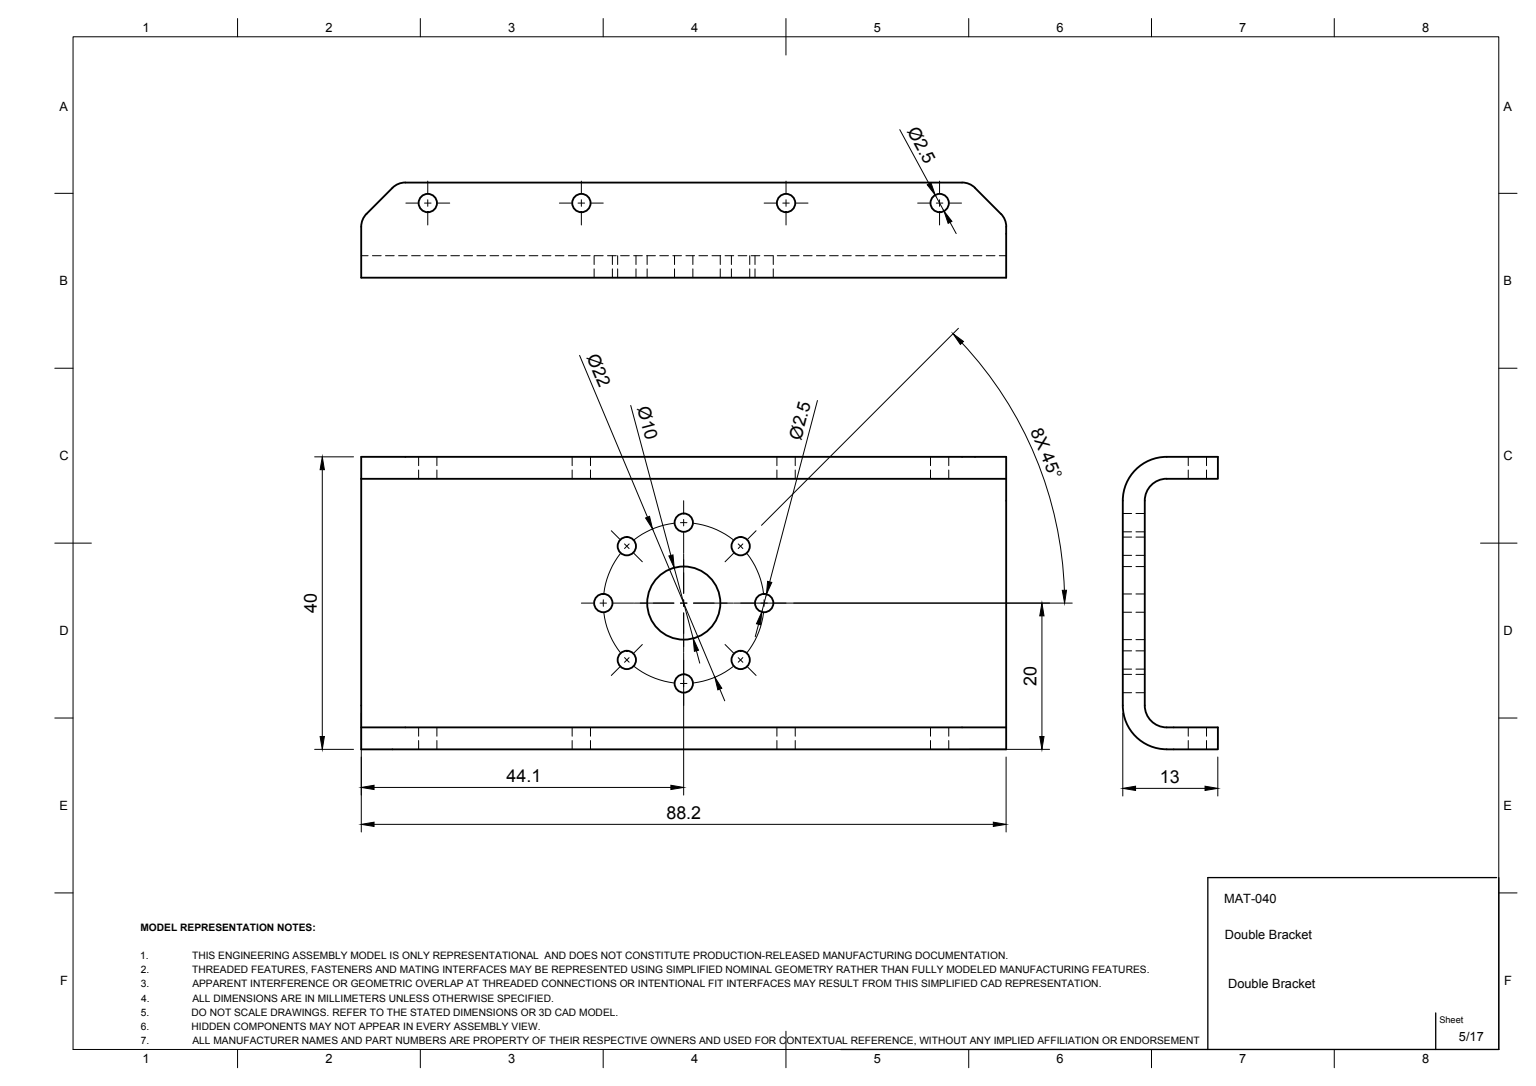
ISO-10303-21;
HEADER;
/* Generated by software containing ST-Developer
 * from STEP Tools, Inc. (www.steptools.com) 
 */

FILE_DESCRIPTION(
/* description */ ('STEP AP214'),
/* implementation_level */ '2;1');

FILE_NAME(
/* name */ 'Double Bracket.step',
/* time_stamp */ '2026-11-14T21:53:28-08:00',
/* author */ (''),
/* organization */ (''),
/* preprocessor_version */ 'ST-DEVELOPER v20.2',
/* originating_system */ 'Autodesk Translation Framework v15.17.0.0',
/* authorisation */ '');

FILE_SCHEMA (('AUTOMOTIVE_DESIGN { 1 0 10303 214 3 1 1 }'));
ENDSEC;

DATA;
#10=MECHANICAL_DESIGN_GEOMETRIC_PRESENTATION_REPRESENTATION('',(#318),#20176);
#294=SHAPE_REPRESENTATION_RELATIONSHIP('SRR','None',#20256,#306);
#306=ADVANCED_BREP_SHAPE_REPRESENTATION('',(#353),#20162);
#318=STYLED_ITEM('',(#20335),#353);
#353=MANIFOLD_SOLID_BREP('Body1',#10944);
#380=FACE_BOUND('',#1518,.T.);
#381=FACE_BOUND('',#1519,.T.);
#382=FACE_BOUND('',#1520,.T.);
#383=FACE_BOUND('',#1521,.T.);
#384=FACE_BOUND('',#1524,.T.);
#385=FACE_BOUND('',#1525,.T.);
#386=FACE_BOUND('',#1526,.T.);
#387=FACE_BOUND('',#1527,.T.);
#388=FACE_BOUND('',#1530,.T.);
#389=FACE_BOUND('',#1531,.T.);
#390=FACE_BOUND('',#1532,.T.);
#391=FACE_BOUND('',#1533,.T.);
#392=FACE_BOUND('',#1534,.T.);
#393=FACE_BOUND('',#1535,.T.);
#394=FACE_BOUND('',#1536,.T.);
#395=FACE_BOUND('',#1537,.T.);
#396=FACE_BOUND('',#1538,.T.);
#397=FACE_BOUND('',#1541,.T.);
#398=FACE_BOUND('',#1542,.T.);
#399=FACE_BOUND('',#1543,.T.);
#400=FACE_BOUND('',#1544,.T.);
#401=FACE_BOUND('',#1547,.T.);
#402=FACE_BOUND('',#1548,.T.);
#403=FACE_BOUND('',#1549,.T.);
#404=FACE_BOUND('',#1550,.T.);
#405=FACE_BOUND('',#1553,.T.);
#406=FACE_BOUND('',#1554,.T.);
#407=FACE_BOUND('',#1555,.T.);
#408=FACE_BOUND('',#1556,.T.);
#409=FACE_BOUND('',#1557,.T.);
#410=FACE_BOUND('',#1558,.T.);
#411=FACE_BOUND('',#1559,.T.);
#412=FACE_BOUND('',#1560,.T.);
#413=FACE_BOUND('',#1561,.T.);
#576=PLANE('',#11157);
#577=PLANE('',#11160);
#578=PLANE('',#11161);
#579=PLANE('',#11164);
#580=PLANE('',#11165);
#581=PLANE('',#11168);
#582=PLANE('',#11169);
#583=PLANE('',#11172);
#584=PLANE('',#11173);
#585=PLANE('',#11178);
#586=PLANE('',#11179);
#587=PLANE('',#11185);
#588=PLANE('',#11187);
#589=PLANE('',#11192);
#590=PLANE('',#11193);
#591=PLANE('',#11199);
#592=PLANE('',#11201);
#593=PLANE('',#11202);
#594=PLANE('',#11203);
#595=PLANE('',#11204);
#596=PLANE('',#11205);
#597=PLANE('',#11206);
#900=FACE_OUTER_BOUND('',#1492,.T.);
#901=FACE_OUTER_BOUND('',#1493,.T.);
#902=FACE_OUTER_BOUND('',#1494,.T.);
#903=FACE_OUTER_BOUND('',#1495,.T.);
#904=FACE_OUTER_BOUND('',#1496,.T.);
#905=FACE_OUTER_BOUND('',#1497,.T.);
#906=FACE_OUTER_BOUND('',#1498,.T.);
#907=FACE_OUTER_BOUND('',#1499,.T.);
#908=FACE_OUTER_BOUND('',#1500,.T.);
#909=FACE_OUTER_BOUND('',#1501,.T.);
#910=FACE_OUTER_BOUND('',#1502,.T.);
#911=FACE_OUTER_BOUND('',#1503,.T.);
#912=FACE_OUTER_BOUND('',#1504,.T.);
#913=FACE_OUTER_BOUND('',#1505,.T.);
#914=FACE_OUTER_BOUND('',#1506,.T.);
#915=FACE_OUTER_BOUND('',#1507,.T.);
#916=FACE_OUTER_BOUND('',#1508,.T.);
#917=FACE_OUTER_BOUND('',#1509,.T.);
#918=FACE_OUTER_BOUND('',#1510,.T.);
#919=FACE_OUTER_BOUND('',#1511,.T.);
#920=FACE_OUTER_BOUND('',#1512,.T.);
#921=FACE_OUTER_BOUND('',#1513,.T.);
#922=FACE_OUTER_BOUND('',#1514,.T.);
#923=FACE_OUTER_BOUND('',#1515,.T.);
#924=FACE_OUTER_BOUND('',#1516,.T.);
#925=FACE_OUTER_BOUND('',#1517,.T.);
#926=FACE_OUTER_BOUND('',#1522,.T.);
#927=FACE_OUTER_BOUND('',#1523,.T.);
#928=FACE_OUTER_BOUND('',#1528,.T.);
#929=FACE_OUTER_BOUND('',#1529,.T.);
#930=FACE_OUTER_BOUND('',#1539,.T.);
#931=FACE_OUTER_BOUND('',#1540,.T.);
#932=FACE_OUTER_BOUND('',#1545,.T.);
#933=FACE_OUTER_BOUND('',#1546,.T.);
#934=FACE_OUTER_BOUND('',#1551,.T.);
#935=FACE_OUTER_BOUND('',#1552,.T.);
#936=FACE_OUTER_BOUND('',#1562,.T.);
#937=FACE_OUTER_BOUND('',#1563,.T.);
#938=FACE_OUTER_BOUND('',#1564,.T.);
#939=FACE_OUTER_BOUND('',#1565,.T.);
#940=FACE_OUTER_BOUND('',#1566,.T.);
#941=FACE_OUTER_BOUND('',#1567,.T.);
#942=FACE_OUTER_BOUND('',#1568,.T.);
#943=FACE_OUTER_BOUND('',#1569,.T.);
#944=FACE_OUTER_BOUND('',#1570,.T.);
#945=FACE_OUTER_BOUND('',#1571,.T.);
#946=FACE_OUTER_BOUND('',#1572,.T.);
#947=FACE_OUTER_BOUND('',#1573,.T.);
#948=FACE_OUTER_BOUND('',#1574,.T.);
#949=FACE_OUTER_BOUND('',#1575,.T.);
#950=FACE_OUTER_BOUND('',#1576,.T.);
#1492=EDGE_LOOP('',(#7183,#7184,#7185,#7186));
#1493=EDGE_LOOP('',(#7187,#7188,#7189,#7190));
#1494=EDGE_LOOP('',(#7191,#7192,#7193,#7194));
#1495=EDGE_LOOP('',(#7195,#7196,#7197,#7198));
#1496=EDGE_LOOP('',(#7199,#7200,#7201,#7202));
#1497=EDGE_LOOP('',(#7203,#7204,#7205,#7206));
#1498=EDGE_LOOP('',(#7207,#7208,#7209,#7210));
#1499=EDGE_LOOP('',(#7211,#7212,#7213,#7214));
#1500=EDGE_LOOP('',(#7215,#7216,#7217,#7218));
#1501=EDGE_LOOP('',(#7219,#7220,#7221,#7222));
#1502=EDGE_LOOP('',(#7223,#7224,#7225,#7226));
#1503=EDGE_LOOP('',(#7227,#7228,#7229,#7230));
#1504=EDGE_LOOP('',(#7231,#7232,#7233,#7234));
#1505=EDGE_LOOP('',(#7235,#7236,#7237,#7238));
#1506=EDGE_LOOP('',(#7239,#7240,#7241,#7242));
#1507=EDGE_LOOP('',(#7243,#7244,#7245,#7246));
#1508=EDGE_LOOP('',(#7247,#7248,#7249,#7250));
#1509=EDGE_LOOP('',(#7251,#7252,#7253,#7254));
#1510=EDGE_LOOP('',(#7255,#7256,#7257,#7258));
#1511=EDGE_LOOP('',(#7259,#7260,#7261,#7262));
#1512=EDGE_LOOP('',(#7263,#7264,#7265,#7266));
#1513=EDGE_LOOP('',(#7267,#7268,#7269,#7270));
#1514=EDGE_LOOP('',(#7271,#7272,#7273,#7274));
#1515=EDGE_LOOP('',(#7275,#7276,#7277,#7278));
#1516=EDGE_LOOP('',(#7279,#7280,#7281,#7282));
#1517=EDGE_LOOP('',(#7283,#7284,#7285,#7286,#7287,#7288,#7289,#7290,#7291,
#7292));
#1518=EDGE_LOOP('',(#7293));
#1519=EDGE_LOOP('',(#7294));
#1520=EDGE_LOOP('',(#7295));
#1521=EDGE_LOOP('',(#7296));
#1522=EDGE_LOOP('',(#7297,#7298,#7299,#7300));
#1523=EDGE_LOOP('',(#7301,#7302,#7303,#7304,#7305,#7306,#7307,#7308,#7309,
#7310));
#1524=EDGE_LOOP('',(#7311));
#1525=EDGE_LOOP('',(#7312));
#1526=EDGE_LOOP('',(#7313));
#1527=EDGE_LOOP('',(#7314));
#1528=EDGE_LOOP('',(#7315,#7316,#7317,#7318));
#1529=EDGE_LOOP('',(#7319,#7320,#7321,#7322));
#1530=EDGE_LOOP('',(#7323));
#1531=EDGE_LOOP('',(#7324));
#1532=EDGE_LOOP('',(#7325));
#1533=EDGE_LOOP('',(#7326));
#1534=EDGE_LOOP('',(#7327));
#1535=EDGE_LOOP('',(#7328));
#1536=EDGE_LOOP('',(#7329));
#1537=EDGE_LOOP('',(#7330));
#1538=EDGE_LOOP('',(#7331));
#1539=EDGE_LOOP('',(#7332,#7333,#7334,#7335));
#1540=EDGE_LOOP('',(#7336,#7337,#7338,#7339,#7340,#7341,#7342,#7343,#7344,
#7345));
#1541=EDGE_LOOP('',(#7346));
#1542=EDGE_LOOP('',(#7347));
#1543=EDGE_LOOP('',(#7348));
#1544=EDGE_LOOP('',(#7349));
#1545=EDGE_LOOP('',(#7350,#7351,#7352,#7353));
#1546=EDGE_LOOP('',(#7354,#7355,#7356,#7357,#7358,#7359,#7360,#7361,#7362,
#7363));
#1547=EDGE_LOOP('',(#7364));
#1548=EDGE_LOOP('',(#7365));
#1549=EDGE_LOOP('',(#7366));
#1550=EDGE_LOOP('',(#7367));
#1551=EDGE_LOOP('',(#7368,#7369,#7370,#7371));
#1552=EDGE_LOOP('',(#7372,#7373,#7374,#7375));
#1553=EDGE_LOOP('',(#7376));
#1554=EDGE_LOOP('',(#7377));
#1555=EDGE_LOOP('',(#7378));
#1556=EDGE_LOOP('',(#7379));
#1557=EDGE_LOOP('',(#7380));
#1558=EDGE_LOOP('',(#7381));
#1559=EDGE_LOOP('',(#7382));
#1560=EDGE_LOOP('',(#7383));
#1561=EDGE_LOOP('',(#7384));
#1562=EDGE_LOOP('',(#7385,#7386,#7387,#7388));
#1563=EDGE_LOOP('',(#7389,#7390,#7391,#7392));
#1564=EDGE_LOOP('',(#7393,#7394,#7395,#7396));
#1565=EDGE_LOOP('',(#7397,#7398,#7399,#7400));
#1566=EDGE_LOOP('',(#7401,#7402,#7403,#7404));
#1567=EDGE_LOOP('',(#7405,#7406,#7407,#7408));
#1568=EDGE_LOOP('',(#7409,#7410,#7411,#7412));
#1569=EDGE_LOOP('',(#7413,#7414,#7415,#7416));
#1570=EDGE_LOOP('',(#7417,#7418,#7419,#7420));
#1571=EDGE_LOOP('',(#7421,#7422,#7423,#7424));
#1572=EDGE_LOOP('',(#7425,#7426,#7427,#7428));
#1573=EDGE_LOOP('',(#7429,#7430,#7431,#7432));
#1574=EDGE_LOOP('',(#7433,#7434,#7435,#7436));
#1575=EDGE_LOOP('',(#7437,#7438,#7439,#7440));
#1576=EDGE_LOOP('',(#7441,#7442,#7443,#7444));
#2280=LINE('',#15428,#3268);
#2281=LINE('',#15434,#3269);
#2282=LINE('',#15440,#3270);
#2283=LINE('',#15446,#3271);
#2284=LINE('',#15452,#3272);
#2285=LINE('',#15458,#3273);
#2286=LINE('',#15464,#3274);
#2287=LINE('',#15470,#3275);
#2288=LINE('',#15476,#3276);
#2289=LINE('',#15482,#3277);
#2290=LINE('',#15488,#3278);
#2291=LINE('',#15494,#3279);
#2292=LINE('',#15500,#3280);
#2293=LINE('',#15506,#3281);
#2294=LINE('',#15512,#3282);
#2295=LINE('',#15518,#3283);
#2296=LINE('',#15524,#3284);
#2297=LINE('',#15529,#3285);
#2298=LINE('',#15533,#3286);
#2299=LINE('',#15537,#3287);
#2300=LINE('',#15539,#3288);
#2301=LINE('',#15540,#3289);
#2302=LINE('',#15544,#3290);
#2303=LINE('',#15548,#3291);
#2304=LINE('',#15552,#3292);
#2305=LINE('',#15554,#3293);
#2306=LINE('',#15555,#3294);
#2307=LINE('',#15559,#3295);
#2308=LINE('',#15564,#3296);
#2309=LINE('',#15566,#3297);
#2310=LINE('',#15567,#3298);
#2311=LINE('',#15571,#3299);
#2312=LINE('',#15575,#3300);
#2313=LINE('',#15578,#3301);
#2314=LINE('',#15579,#3302);
#2315=LINE('',#15583,#3303);
#2316=LINE('',#15585,#3304);
#2317=LINE('',#15587,#3305);
#2318=LINE('',#15591,#3306);
#2319=LINE('',#15595,#3307);
#2320=LINE('',#15600,#3308);
#2321=LINE('',#15601,#3309);
#2322=LINE('',#15602,#3310);
#2323=LINE('',#15607,#3311);
#2324=LINE('',#15612,#3312);
#2325=LINE('',#15615,#3313);
#2326=LINE('',#15616,#3314);
#2327=LINE('',#15618,#3315);
#2328=LINE('',#15620,#3316);
#2329=LINE('',#15622,#3317);
#2330=LINE('',#15627,#3318);
#2331=LINE('',#15631,#3319);
#2332=LINE('',#15635,#3320);
#2333=LINE('',#15638,#3321);
#2334=LINE('',#15641,#3322);
#2335=LINE('',#15643,#3323);
#2336=LINE('',#15644,#3324);
#2337=LINE('',#15648,#3325);
#2338=LINE('',#15650,#3326);
#2339=LINE('',#15652,#3327);
#2340=LINE('',#15656,#3328);
#2341=LINE('',#15660,#3329);
#2342=LINE('',#15662,#3330);
#2343=LINE('',#15665,#3331);
#2344=LINE('',#15667,#3332);
#2345=LINE('',#15669,#3333);
#2346=LINE('',#15670,#3334);
#2347=LINE('',#15672,#3335);
#2348=LINE('',#15673,#3336);
#2349=LINE('',#15675,#3337);
#2350=LINE('',#15676,#3338);
#2351=LINE('',#15678,#3339);
#2352=LINE('',#15679,#3340);
#3268=VECTOR('',#12222,1.25);
#3269=VECTOR('',#12229,1.25);
#3270=VECTOR('',#12236,1.25);
#3271=VECTOR('',#12243,1.25);
#3272=VECTOR('',#12250,1.25);
#3273=VECTOR('',#12257,1.25);
#3274=VECTOR('',#12264,1.25);
#3275=VECTOR('',#12271,1.25);
#3276=VECTOR('',#12278,1.25);
#3277=VECTOR('',#12285,1.25);
#3278=VECTOR('',#12292,1.25);
#3279=VECTOR('',#12299,1.25);
#3280=VECTOR('',#12306,1.25);
#3281=VECTOR('',#12313,1.25);
#3282=VECTOR('',#12320,1.25);
#3283=VECTOR('',#12327,1.25);
#3284=VECTOR('',#12334,5.);
#3285=VECTOR('',#12339,1000.);
#3286=VECTOR('',#12342,1000.);
#3287=VECTOR('',#12347,1000.);
#3288=VECTOR('',#12348,1000.);
#3289=VECTOR('',#12349,1000.);
#3290=VECTOR('',#12352,1000.);
#3291=VECTOR('',#12355,1000.);
#3292=VECTOR('',#12360,1000.);
#3293=VECTOR('',#12361,1000.);
#3294=VECTOR('',#12362,1000.);
#3295=VECTOR('',#12365,1000.);
#3296=VECTOR('',#12372,1000.);
#3297=VECTOR('',#12373,1000.);
#3298=VECTOR('',#12374,1000.);
#3299=VECTOR('',#12377,1000.);
#3300=VECTOR('',#12380,1000.);
#3301=VECTOR('',#12385,1000.);
#3302=VECTOR('',#12386,1000.);
#3303=VECTOR('',#12389,1000.);
#3304=VECTOR('',#12392,1000.);
#3305=VECTOR('',#12393,1000.);
#3306=VECTOR('',#12396,1000.);
#3307=VECTOR('',#12399,1000.);
#3308=VECTOR('',#12404,1000.);
#3309=VECTOR('',#12405,1000.);
#3310=VECTOR('',#12406,1000.);
#3311=VECTOR('',#12411,1000.);
#3312=VECTOR('',#12416,1000.);
#3313=VECTOR('',#12419,1000.);
#3314=VECTOR('',#12420,1000.);
#3315=VECTOR('',#12423,1000.);
#3316=VECTOR('',#12426,1000.);
#3317=VECTOR('',#12429,1000.);
#3318=VECTOR('',#12434,1000.);
#3319=VECTOR('',#12437,1000.);
#3320=VECTOR('',#12440,1000.);
#3321=VECTOR('',#12443,1000.);
#3322=VECTOR('',#12446,1000.);
#3323=VECTOR('',#12447,1000.);
#3324=VECTOR('',#12448,1000.);
#3325=VECTOR('',#12451,1000.);
#3326=VECTOR('',#12454,1000.);
#3327=VECTOR('',#12455,1000.);
#3328=VECTOR('',#12458,1000.);
#3329=VECTOR('',#12465,1000.);
#3330=VECTOR('',#12468,1000.);
#3331=VECTOR('',#12473,1000.);
#3332=VECTOR('',#12476,1000.);
#3333=VECTOR('',#12479,1000.);
#3334=VECTOR('',#12480,1000.);
#3335=VECTOR('',#12483,1000.);
#3336=VECTOR('',#12484,1000.);
#3337=VECTOR('',#12487,1000.);
#3338=VECTOR('',#12488,1000.);
#3339=VECTOR('',#12491,1000.);
#3340=VECTOR('',#12492,1000.);
#4256=CIRCLE('',#11107,1.25);
#4257=CIRCLE('',#11108,1.25);
#4258=CIRCLE('',#11110,1.25);
#4259=CIRCLE('',#11111,1.25);
#4260=CIRCLE('',#11113,1.25);
#4261=CIRCLE('',#11114,1.25);
#4262=CIRCLE('',#11116,1.25);
#4263=CIRCLE('',#11117,1.25);
#4264=CIRCLE('',#11119,1.25);
#4265=CIRCLE('',#11120,1.25);
#4266=CIRCLE('',#11122,1.25);
#4267=CIRCLE('',#11123,1.25);
#4268=CIRCLE('',#11125,1.25);
#4269=CIRCLE('',#11126,1.25);
#4270=CIRCLE('',#11128,1.25);
#4271=CIRCLE('',#11129,1.25);
#4272=CIRCLE('',#11131,1.24999999999999);
#4273=CIRCLE('',#11132,1.25);
#4274=CIRCLE('',#11134,1.24999999999999);
#4275=CIRCLE('',#11135,1.25);
#4276=CIRCLE('',#11137,1.24999999999999);
#4277=CIRCLE('',#11138,1.25);
#4278=CIRCLE('',#11140,1.24999999999999);
#4279=CIRCLE('',#11141,1.25);
#4280=CIRCLE('',#11143,1.24999999999999);
#4281=CIRCLE('',#11144,1.25);
#4282=CIRCLE('',#11146,1.25);
#4283=CIRCLE('',#11147,1.25);
#4284=CIRCLE('',#11149,1.25000000000001);
#4285=CIRCLE('',#11150,1.25);
#4286=CIRCLE('',#11152,1.25);
#4287=CIRCLE('',#11153,1.25);
#4288=CIRCLE('',#11155,5.);
#4289=CIRCLE('',#11156,5.);
#4290=CIRCLE('',#11158,3.);
#4291=CIRCLE('',#11159,6.);
#4292=CIRCLE('',#11162,3.);
#4293=CIRCLE('',#11163,6.);
#4294=CIRCLE('',#11166,3.);
#4295=CIRCLE('',#11167,6.);
#4296=CIRCLE('',#11170,3.);
#4297=CIRCLE('',#11171,6.);
#4298=CIRCLE('',#11174,2.5);
#4299=CIRCLE('',#11175,2.5);
#4300=CIRCLE('',#11176,2.5);
#4301=CIRCLE('',#11177,2.5);
#4302=CIRCLE('',#11180,2.5);
#4303=CIRCLE('',#11181,2.5);
#4304=CIRCLE('',#11182,2.5);
#4305=CIRCLE('',#11183,2.5);
#4306=CIRCLE('',#11188,2.5);
#4307=CIRCLE('',#11189,2.5);
#4308=CIRCLE('',#11190,2.5);
#4309=CIRCLE('',#11191,2.5);
#4310=CIRCLE('',#11194,2.5);
#4311=CIRCLE('',#11195,2.5);
#4312=CIRCLE('',#11196,2.5);
#4313=CIRCLE('',#11197,2.5);
#4727=VERTEX_POINT('',#15425);
#4728=VERTEX_POINT('',#15427);
#4729=VERTEX_POINT('',#15431);
#4730=VERTEX_POINT('',#15433);
#4731=VERTEX_POINT('',#15437);
#4732=VERTEX_POINT('',#15439);
#4733=VERTEX_POINT('',#15443);
#4734=VERTEX_POINT('',#15445);
#4735=VERTEX_POINT('',#15449);
#4736=VERTEX_POINT('',#15451);
#4737=VERTEX_POINT('',#15455);
#4738=VERTEX_POINT('',#15457);
#4739=VERTEX_POINT('',#15461);
#4740=VERTEX_POINT('',#15463);
#4741=VERTEX_POINT('',#15467);
#4742=VERTEX_POINT('',#15469);
#4743=VERTEX_POINT('',#15473);
#4744=VERTEX_POINT('',#15475);
#4745=VERTEX_POINT('',#15479);
#4746=VERTEX_POINT('',#15481);
#4747=VERTEX_POINT('',#15485);
#4748=VERTEX_POINT('',#15487);
#4749=VERTEX_POINT('',#15491);
#4750=VERTEX_POINT('',#15493);
#4751=VERTEX_POINT('',#15497);
#4752=VERTEX_POINT('',#15499);
#4753=VERTEX_POINT('',#15503);
#4754=VERTEX_POINT('',#15505);
#4755=VERTEX_POINT('',#15509);
#4756=VERTEX_POINT('',#15511);
#4757=VERTEX_POINT('',#15515);
#4758=VERTEX_POINT('',#15517);
#4759=VERTEX_POINT('',#15521);
#4760=VERTEX_POINT('',#15523);
#4761=VERTEX_POINT('',#15527);
#4762=VERTEX_POINT('',#15528);
#4763=VERTEX_POINT('',#15530);
#4764=VERTEX_POINT('',#15532);
#4765=VERTEX_POINT('',#15536);
#4766=VERTEX_POINT('',#15538);
#4767=VERTEX_POINT('',#15542);
#4768=VERTEX_POINT('',#15543);
#4769=VERTEX_POINT('',#15545);
#4770=VERTEX_POINT('',#15547);
#4771=VERTEX_POINT('',#15551);
#4772=VERTEX_POINT('',#15553);
#4773=VERTEX_POINT('',#15557);
#4774=VERTEX_POINT('',#15558);
#4775=VERTEX_POINT('',#15563);
#4776=VERTEX_POINT('',#15565);
#4777=VERTEX_POINT('',#15569);
#4778=VERTEX_POINT('',#15570);
#4779=VERTEX_POINT('',#15572);
#4780=VERTEX_POINT('',#15574);
#4781=VERTEX_POINT('',#15581);
#4782=VERTEX_POINT('',#15582);
#4783=VERTEX_POINT('',#15586);
#4784=VERTEX_POINT('',#15588);
#4785=VERTEX_POINT('',#15590);
#4786=VERTEX_POINT('',#15592);
#4787=VERTEX_POINT('',#15594);
#4788=VERTEX_POINT('',#15598);
#4789=VERTEX_POINT('',#15599);
#4790=VERTEX_POINT('',#15604);
#4791=VERTEX_POINT('',#15606);
#4792=VERTEX_POINT('',#15609);
#4793=VERTEX_POINT('',#15611);
#4794=VERTEX_POINT('',#15613);
#4795=VERTEX_POINT('',#15624);
#4796=VERTEX_POINT('',#15626);
#4797=VERTEX_POINT('',#15628);
#4798=VERTEX_POINT('',#15630);
#4799=VERTEX_POINT('',#15632);
#4800=VERTEX_POINT('',#15634);
#4801=VERTEX_POINT('',#15636);
#4802=VERTEX_POINT('',#15640);
#4803=VERTEX_POINT('',#15642);
#4804=VERTEX_POINT('',#15646);
#4805=VERTEX_POINT('',#15647);
#4806=VERTEX_POINT('',#15651);
#4807=VERTEX_POINT('',#15653);
#4808=VERTEX_POINT('',#15655);
#5694=EDGE_CURVE('',#4727,#4727,#4256,.T.);
#5695=EDGE_CURVE('',#4727,#4728,#2280,.T.);
#5696=EDGE_CURVE('',#4728,#4728,#4257,.T.);
#5697=EDGE_CURVE('',#4729,#4729,#4258,.T.);
#5698=EDGE_CURVE('',#4729,#4730,#2281,.T.);
#5699=EDGE_CURVE('',#4730,#4730,#4259,.T.);
#5700=EDGE_CURVE('',#4731,#4731,#4260,.T.);
#5701=EDGE_CURVE('',#4731,#4732,#2282,.T.);
#5702=EDGE_CURVE('',#4732,#4732,#4261,.T.);
#5703=EDGE_CURVE('',#4733,#4733,#4262,.T.);
#5704=EDGE_CURVE('',#4733,#4734,#2283,.T.);
#5705=EDGE_CURVE('',#4734,#4734,#4263,.T.);
#5706=EDGE_CURVE('',#4735,#4735,#4264,.T.);
#5707=EDGE_CURVE('',#4735,#4736,#2284,.T.);
#5708=EDGE_CURVE('',#4736,#4736,#4265,.T.);
#5709=EDGE_CURVE('',#4737,#4737,#4266,.T.);
#5710=EDGE_CURVE('',#4737,#4738,#2285,.T.);
#5711=EDGE_CURVE('',#4738,#4738,#4267,.T.);
#5712=EDGE_CURVE('',#4739,#4739,#4268,.T.);
#5713=EDGE_CURVE('',#4739,#4740,#2286,.T.);
#5714=EDGE_CURVE('',#4740,#4740,#4269,.T.);
#5715=EDGE_CURVE('',#4741,#4741,#4270,.T.);
#5716=EDGE_CURVE('',#4741,#4742,#2287,.T.);
#5717=EDGE_CURVE('',#4742,#4742,#4271,.T.);
#5718=EDGE_CURVE('',#4743,#4743,#4272,.T.);
#5719=EDGE_CURVE('',#4743,#4744,#2288,.T.);
#5720=EDGE_CURVE('',#4744,#4744,#4273,.T.);
#5721=EDGE_CURVE('',#4745,#4745,#4274,.T.);
#5722=EDGE_CURVE('',#4745,#4746,#2289,.T.);
#5723=EDGE_CURVE('',#4746,#4746,#4275,.T.);
#5724=EDGE_CURVE('',#4747,#4747,#4276,.T.);
#5725=EDGE_CURVE('',#4747,#4748,#2290,.T.);
#5726=EDGE_CURVE('',#4748,#4748,#4277,.T.);
#5727=EDGE_CURVE('',#4749,#4749,#4278,.T.);
#5728=EDGE_CURVE('',#4749,#4750,#2291,.T.);
#5729=EDGE_CURVE('',#4750,#4750,#4279,.T.);
#5730=EDGE_CURVE('',#4751,#4751,#4280,.T.);
#5731=EDGE_CURVE('',#4751,#4752,#2292,.T.);
#5732=EDGE_CURVE('',#4752,#4752,#4281,.T.);
#5733=EDGE_CURVE('',#4753,#4753,#4282,.T.);
#5734=EDGE_CURVE('',#4753,#4754,#2293,.T.);
#5735=EDGE_CURVE('',#4754,#4754,#4283,.T.);
#5736=EDGE_CURVE('',#4755,#4755,#4284,.T.);
#5737=EDGE_CURVE('',#4755,#4756,#2294,.T.);
#5738=EDGE_CURVE('',#4756,#4756,#4285,.T.);
#5739=EDGE_CURVE('',#4757,#4757,#4286,.T.);
#5740=EDGE_CURVE('',#4757,#4758,#2295,.T.);
#5741=EDGE_CURVE('',#4758,#4758,#4287,.T.);
#5742=EDGE_CURVE('',#4759,#4759,#4288,.T.);
#5743=EDGE_CURVE('',#4759,#4760,#2296,.T.);
#5744=EDGE_CURVE('',#4760,#4760,#4289,.T.);
#5745=EDGE_CURVE('',#4761,#4762,#2297,.T.);
#5746=EDGE_CURVE('',#4763,#4761,#4290,.T.);
#5747=EDGE_CURVE('',#4764,#4763,#2298,.T.);
#5748=EDGE_CURVE('',#4764,#4762,#4291,.T.);
#5749=EDGE_CURVE('',#4761,#4765,#2299,.T.);
#5750=EDGE_CURVE('',#4762,#4766,#2300,.T.);
#5751=EDGE_CURVE('',#4766,#4765,#2301,.T.);
#5752=EDGE_CURVE('',#4767,#4768,#2302,.T.);
#5753=EDGE_CURVE('',#4767,#4769,#4292,.T.);
#5754=EDGE_CURVE('',#4770,#4769,#2303,.T.);
#5755=EDGE_CURVE('',#4768,#4770,#4293,.T.);
#5756=EDGE_CURVE('',#4771,#4768,#2304,.T.);
#5757=EDGE_CURVE('',#4771,#4772,#2305,.T.);
#5758=EDGE_CURVE('',#4772,#4767,#2306,.T.);
#5759=EDGE_CURVE('',#4773,#4774,#2307,.T.);
#5760=EDGE_CURVE('',#4765,#4773,#4294,.T.);
#5761=EDGE_CURVE('',#4766,#4774,#4295,.T.);
#5762=EDGE_CURVE('',#4774,#4775,#2308,.T.);
#5763=EDGE_CURVE('',#4775,#4776,#2309,.T.);
#5764=EDGE_CURVE('',#4773,#4776,#2310,.T.);
#5765=EDGE_CURVE('',#4777,#4778,#2311,.T.);
#5766=EDGE_CURVE('',#4777,#4779,#4296,.T.);
#5767=EDGE_CURVE('',#4780,#4779,#2312,.T.);
#5768=EDGE_CURVE('',#4778,#4780,#4297,.T.);
#5769=EDGE_CURVE('',#4769,#4777,#2313,.T.);
#5770=EDGE_CURVE('',#4770,#4778,#2314,.T.);
#5771=EDGE_CURVE('',#4781,#4782,#2315,.T.);
#5772=EDGE_CURVE('',#4782,#4775,#4298,.T.);
#5773=EDGE_CURVE('',#4774,#4780,#2316,.T.);
#5774=EDGE_CURVE('',#4780,#4783,#2317,.T.);
#5775=EDGE_CURVE('',#4783,#4784,#4299,.T.);
#5776=EDGE_CURVE('',#4784,#4785,#2318,.T.);
#5777=EDGE_CURVE('',#4785,#4786,#4300,.T.);
#5778=EDGE_CURVE('',#4787,#4786,#2319,.T.);
#5779=EDGE_CURVE('',#4787,#4781,#4301,.T.);
#5780=EDGE_CURVE('',#4788,#4789,#2320,.T.);
#5781=EDGE_CURVE('',#4788,#4787,#2321,.T.);
#5782=EDGE_CURVE('',#4786,#4789,#2322,.T.);
#5783=EDGE_CURVE('',#4776,#4790,#4302,.T.);
#5784=EDGE_CURVE('',#4790,#4791,#2323,.T.);
#5785=EDGE_CURVE('',#4791,#4788,#4303,.T.);
#5786=EDGE_CURVE('',#4789,#4792,#4304,.T.);
#5787=EDGE_CURVE('',#4792,#4793,#2324,.T.);
#5788=EDGE_CURVE('',#4793,#4794,#4305,.T.);
#5789=EDGE_CURVE('',#4779,#4794,#2325,.T.);
#5790=EDGE_CURVE('',#4773,#4779,#2326,.T.);
#5791=EDGE_CURVE('',#4765,#4777,#2327,.T.);
#5792=EDGE_CURVE('',#4761,#4769,#2328,.T.);
#5793=EDGE_CURVE('',#4763,#4767,#2329,.T.);
#5794=EDGE_CURVE('',#4772,#4795,#4306,.T.);
#5795=EDGE_CURVE('',#4795,#4796,#2330,.T.);
#5796=EDGE_CURVE('',#4796,#4797,#4307,.T.);
#5797=EDGE_CURVE('',#4798,#4797,#2331,.T.);
#5798=EDGE_CURVE('',#4798,#4799,#4308,.T.);
#5799=EDGE_CURVE('',#4799,#4800,#2332,.T.);
#5800=EDGE_CURVE('',#4800,#4801,#4309,.T.);
#5801=EDGE_CURVE('',#4801,#4763,#2333,.T.);
#5802=EDGE_CURVE('',#4797,#4802,#2334,.T.);
#5803=EDGE_CURVE('',#4803,#4802,#2335,.T.);
#5804=EDGE_CURVE('',#4803,#4798,#2336,.T.);
#5805=EDGE_CURVE('',#4804,#4805,#2337,.T.);
#5806=EDGE_CURVE('',#4805,#4771,#4310,.T.);
#5807=EDGE_CURVE('',#4764,#4768,#2338,.T.);
#5808=EDGE_CURVE('',#4806,#4764,#2339,.T.);
#5809=EDGE_CURVE('',#4806,#4807,#4311,.T.);
#5810=EDGE_CURVE('',#4807,#4808,#2340,.T.);
#5811=EDGE_CURVE('',#4808,#4803,#4312,.T.);
#5812=EDGE_CURVE('',#4802,#4804,#4313,.T.);
#5813=EDGE_CURVE('',#4762,#4770,#2341,.T.);
#5814=EDGE_CURVE('',#4766,#4778,#2342,.T.);
#5815=EDGE_CURVE('',#4801,#4806,#2343,.T.);
#5816=EDGE_CURVE('',#4794,#4783,#2344,.T.);
#5817=EDGE_CURVE('',#4792,#4785,#2345,.T.);
#5818=EDGE_CURVE('',#4784,#4793,#2346,.T.);
#5819=EDGE_CURVE('',#4795,#4805,#2347,.T.);
#5820=EDGE_CURVE('',#4804,#4796,#2348,.T.);
#5821=EDGE_CURVE('',#4790,#4782,#2349,.T.);
#5822=EDGE_CURVE('',#4781,#4791,#2350,.T.);
#5823=EDGE_CURVE('',#4807,#4800,#2351,.T.);
#5824=EDGE_CURVE('',#4799,#4808,#2352,.T.);
#7183=ORIENTED_EDGE('',*,*,#5694,.F.);
#7184=ORIENTED_EDGE('',*,*,#5695,.T.);
#7185=ORIENTED_EDGE('',*,*,#5696,.T.);
#7186=ORIENTED_EDGE('',*,*,#5695,.F.);
#7187=ORIENTED_EDGE('',*,*,#5697,.T.);
#7188=ORIENTED_EDGE('',*,*,#5698,.T.);
#7189=ORIENTED_EDGE('',*,*,#5699,.T.);
#7190=ORIENTED_EDGE('',*,*,#5698,.F.);
#7191=ORIENTED_EDGE('',*,*,#5700,.F.);
#7192=ORIENTED_EDGE('',*,*,#5701,.T.);
#7193=ORIENTED_EDGE('',*,*,#5702,.T.);
#7194=ORIENTED_EDGE('',*,*,#5701,.F.);
#7195=ORIENTED_EDGE('',*,*,#5703,.T.);
#7196=ORIENTED_EDGE('',*,*,#5704,.T.);
#7197=ORIENTED_EDGE('',*,*,#5705,.T.);
#7198=ORIENTED_EDGE('',*,*,#5704,.F.);
#7199=ORIENTED_EDGE('',*,*,#5706,.F.);
#7200=ORIENTED_EDGE('',*,*,#5707,.T.);
#7201=ORIENTED_EDGE('',*,*,#5708,.T.);
#7202=ORIENTED_EDGE('',*,*,#5707,.F.);
#7203=ORIENTED_EDGE('',*,*,#5709,.T.);
#7204=ORIENTED_EDGE('',*,*,#5710,.T.);
#7205=ORIENTED_EDGE('',*,*,#5711,.T.);
#7206=ORIENTED_EDGE('',*,*,#5710,.F.);
#7207=ORIENTED_EDGE('',*,*,#5712,.F.);
#7208=ORIENTED_EDGE('',*,*,#5713,.T.);
#7209=ORIENTED_EDGE('',*,*,#5714,.T.);
#7210=ORIENTED_EDGE('',*,*,#5713,.F.);
#7211=ORIENTED_EDGE('',*,*,#5715,.T.);
#7212=ORIENTED_EDGE('',*,*,#5716,.T.);
#7213=ORIENTED_EDGE('',*,*,#5717,.T.);
#7214=ORIENTED_EDGE('',*,*,#5716,.F.);
#7215=ORIENTED_EDGE('',*,*,#5718,.T.);
#7216=ORIENTED_EDGE('',*,*,#5719,.T.);
#7217=ORIENTED_EDGE('',*,*,#5720,.T.);
#7218=ORIENTED_EDGE('',*,*,#5719,.F.);
#7219=ORIENTED_EDGE('',*,*,#5721,.T.);
#7220=ORIENTED_EDGE('',*,*,#5722,.T.);
#7221=ORIENTED_EDGE('',*,*,#5723,.T.);
#7222=ORIENTED_EDGE('',*,*,#5722,.F.);
#7223=ORIENTED_EDGE('',*,*,#5724,.T.);
#7224=ORIENTED_EDGE('',*,*,#5725,.T.);
#7225=ORIENTED_EDGE('',*,*,#5726,.T.);
#7226=ORIENTED_EDGE('',*,*,#5725,.F.);
#7227=ORIENTED_EDGE('',*,*,#5727,.T.);
#7228=ORIENTED_EDGE('',*,*,#5728,.T.);
#7229=ORIENTED_EDGE('',*,*,#5729,.T.);
#7230=ORIENTED_EDGE('',*,*,#5728,.F.);
#7231=ORIENTED_EDGE('',*,*,#5730,.T.);
#7232=ORIENTED_EDGE('',*,*,#5731,.T.);
#7233=ORIENTED_EDGE('',*,*,#5732,.T.);
#7234=ORIENTED_EDGE('',*,*,#5731,.F.);
#7235=ORIENTED_EDGE('',*,*,#5733,.T.);
#7236=ORIENTED_EDGE('',*,*,#5734,.T.);
#7237=ORIENTED_EDGE('',*,*,#5735,.T.);
#7238=ORIENTED_EDGE('',*,*,#5734,.F.);
#7239=ORIENTED_EDGE('',*,*,#5736,.T.);
#7240=ORIENTED_EDGE('',*,*,#5737,.T.);
#7241=ORIENTED_EDGE('',*,*,#5738,.T.);
#7242=ORIENTED_EDGE('',*,*,#5737,.F.);
#7243=ORIENTED_EDGE('',*,*,#5739,.T.);
#7244=ORIENTED_EDGE('',*,*,#5740,.T.);
#7245=ORIENTED_EDGE('',*,*,#5741,.T.);
#7246=ORIENTED_EDGE('',*,*,#5740,.F.);
#7247=ORIENTED_EDGE('',*,*,#5742,.T.);
#7248=ORIENTED_EDGE('',*,*,#5743,.T.);
#7249=ORIENTED_EDGE('',*,*,#5744,.T.);
#7250=ORIENTED_EDGE('',*,*,#5743,.F.);
#7251=ORIENTED_EDGE('',*,*,#5745,.F.);
#7252=ORIENTED_EDGE('',*,*,#5746,.F.);
#7253=ORIENTED_EDGE('',*,*,#5747,.F.);
#7254=ORIENTED_EDGE('',*,*,#5748,.T.);
#7255=ORIENTED_EDGE('',*,*,#5749,.F.);
#7256=ORIENTED_EDGE('',*,*,#5745,.T.);
#7257=ORIENTED_EDGE('',*,*,#5750,.T.);
#7258=ORIENTED_EDGE('',*,*,#5751,.T.);
#7259=ORIENTED_EDGE('',*,*,#5752,.F.);
#7260=ORIENTED_EDGE('',*,*,#5753,.T.);
#7261=ORIENTED_EDGE('',*,*,#5754,.F.);
#7262=ORIENTED_EDGE('',*,*,#5755,.F.);
#7263=ORIENTED_EDGE('',*,*,#5756,.F.);
#7264=ORIENTED_EDGE('',*,*,#5757,.T.);
#7265=ORIENTED_EDGE('',*,*,#5758,.T.);
#7266=ORIENTED_EDGE('',*,*,#5752,.T.);
#7267=ORIENTED_EDGE('',*,*,#5759,.F.);
#7268=ORIENTED_EDGE('',*,*,#5760,.F.);
#7269=ORIENTED_EDGE('',*,*,#5751,.F.);
#7270=ORIENTED_EDGE('',*,*,#5761,.T.);
#7271=ORIENTED_EDGE('',*,*,#5762,.T.);
#7272=ORIENTED_EDGE('',*,*,#5763,.T.);
#7273=ORIENTED_EDGE('',*,*,#5764,.F.);
#7274=ORIENTED_EDGE('',*,*,#5759,.T.);
#7275=ORIENTED_EDGE('',*,*,#5765,.F.);
#7276=ORIENTED_EDGE('',*,*,#5766,.T.);
#7277=ORIENTED_EDGE('',*,*,#5767,.F.);
#7278=ORIENTED_EDGE('',*,*,#5768,.F.);
#7279=ORIENTED_EDGE('',*,*,#5769,.T.);
#7280=ORIENTED_EDGE('',*,*,#5765,.T.);
#7281=ORIENTED_EDGE('',*,*,#5770,.F.);
#7282=ORIENTED_EDGE('',*,*,#5754,.T.);
#7283=ORIENTED_EDGE('',*,*,#5771,.T.);
#7284=ORIENTED_EDGE('',*,*,#5772,.T.);
#7285=ORIENTED_EDGE('',*,*,#5762,.F.);
#7286=ORIENTED_EDGE('',*,*,#5773,.T.);
#7287=ORIENTED_EDGE('',*,*,#5774,.T.);
#7288=ORIENTED_EDGE('',*,*,#5775,.T.);
#7289=ORIENTED_EDGE('',*,*,#5776,.T.);
#7290=ORIENTED_EDGE('',*,*,#5777,.T.);
#7291=ORIENTED_EDGE('',*,*,#5778,.F.);
#7292=ORIENTED_EDGE('',*,*,#5779,.T.);
#7293=ORIENTED_EDGE('',*,*,#5694,.T.);
#7294=ORIENTED_EDGE('',*,*,#5700,.T.);
#7295=ORIENTED_EDGE('',*,*,#5706,.T.);
#7296=ORIENTED_EDGE('',*,*,#5712,.T.);
#7297=ORIENTED_EDGE('',*,*,#5780,.F.);
#7298=ORIENTED_EDGE('',*,*,#5781,.T.);
#7299=ORIENTED_EDGE('',*,*,#5778,.T.);
#7300=ORIENTED_EDGE('',*,*,#5782,.T.);
#7301=ORIENTED_EDGE('',*,*,#5764,.T.);
#7302=ORIENTED_EDGE('',*,*,#5783,.T.);
#7303=ORIENTED_EDGE('',*,*,#5784,.T.);
#7304=ORIENTED_EDGE('',*,*,#5785,.T.);
#7305=ORIENTED_EDGE('',*,*,#5780,.T.);
#7306=ORIENTED_EDGE('',*,*,#5786,.T.);
#7307=ORIENTED_EDGE('',*,*,#5787,.T.);
#7308=ORIENTED_EDGE('',*,*,#5788,.T.);
#7309=ORIENTED_EDGE('',*,*,#5789,.F.);
#7310=ORIENTED_EDGE('',*,*,#5790,.F.);
#7311=ORIENTED_EDGE('',*,*,#5696,.F.);
#7312=ORIENTED_EDGE('',*,*,#5702,.F.);
#7313=ORIENTED_EDGE('',*,*,#5708,.F.);
#7314=ORIENTED_EDGE('',*,*,#5714,.F.);
#7315=ORIENTED_EDGE('',*,*,#5766,.F.);
#7316=ORIENTED_EDGE('',*,*,#5791,.F.);
#7317=ORIENTED_EDGE('',*,*,#5760,.T.);
#7318=ORIENTED_EDGE('',*,*,#5790,.T.);
#7319=ORIENTED_EDGE('',*,*,#5769,.F.);
#7320=ORIENTED_EDGE('',*,*,#5792,.F.);
#7321=ORIENTED_EDGE('',*,*,#5749,.T.);
#7322=ORIENTED_EDGE('',*,*,#5791,.T.);
#7323=ORIENTED_EDGE('',*,*,#5718,.F.);
#7324=ORIENTED_EDGE('',*,*,#5721,.F.);
#7325=ORIENTED_EDGE('',*,*,#5724,.F.);
#7326=ORIENTED_EDGE('',*,*,#5727,.F.);
#7327=ORIENTED_EDGE('',*,*,#5730,.F.);
#7328=ORIENTED_EDGE('',*,*,#5733,.F.);
#7329=ORIENTED_EDGE('',*,*,#5736,.F.);
#7330=ORIENTED_EDGE('',*,*,#5739,.F.);
#7331=ORIENTED_EDGE('',*,*,#5742,.F.);
#7332=ORIENTED_EDGE('',*,*,#5753,.F.);
#7333=ORIENTED_EDGE('',*,*,#5793,.F.);
#7334=ORIENTED_EDGE('',*,*,#5746,.T.);
#7335=ORIENTED_EDGE('',*,*,#5792,.T.);
#7336=ORIENTED_EDGE('',*,*,#5758,.F.);
#7337=ORIENTED_EDGE('',*,*,#5794,.T.);
#7338=ORIENTED_EDGE('',*,*,#5795,.T.);
#7339=ORIENTED_EDGE('',*,*,#5796,.T.);
#7340=ORIENTED_EDGE('',*,*,#5797,.F.);
#7341=ORIENTED_EDGE('',*,*,#5798,.T.);
#7342=ORIENTED_EDGE('',*,*,#5799,.T.);
#7343=ORIENTED_EDGE('',*,*,#5800,.T.);
#7344=ORIENTED_EDGE('',*,*,#5801,.T.);
#7345=ORIENTED_EDGE('',*,*,#5793,.T.);
#7346=ORIENTED_EDGE('',*,*,#5697,.F.);
#7347=ORIENTED_EDGE('',*,*,#5703,.F.);
#7348=ORIENTED_EDGE('',*,*,#5709,.F.);
#7349=ORIENTED_EDGE('',*,*,#5715,.F.);
#7350=ORIENTED_EDGE('',*,*,#5797,.T.);
#7351=ORIENTED_EDGE('',*,*,#5802,.T.);
#7352=ORIENTED_EDGE('',*,*,#5803,.F.);
#7353=ORIENTED_EDGE('',*,*,#5804,.T.);
#7354=ORIENTED_EDGE('',*,*,#5805,.T.);
#7355=ORIENTED_EDGE('',*,*,#5806,.T.);
#7356=ORIENTED_EDGE('',*,*,#5756,.T.);
#7357=ORIENTED_EDGE('',*,*,#5807,.F.);
#7358=ORIENTED_EDGE('',*,*,#5808,.F.);
#7359=ORIENTED_EDGE('',*,*,#5809,.T.);
#7360=ORIENTED_EDGE('',*,*,#5810,.T.);
#7361=ORIENTED_EDGE('',*,*,#5811,.T.);
#7362=ORIENTED_EDGE('',*,*,#5803,.T.);
#7363=ORIENTED_EDGE('',*,*,#5812,.T.);
#7364=ORIENTED_EDGE('',*,*,#5699,.F.);
#7365=ORIENTED_EDGE('',*,*,#5705,.F.);
#7366=ORIENTED_EDGE('',*,*,#5711,.F.);
#7367=ORIENTED_EDGE('',*,*,#5717,.F.);
#7368=ORIENTED_EDGE('',*,*,#5755,.T.);
#7369=ORIENTED_EDGE('',*,*,#5813,.F.);
#7370=ORIENTED_EDGE('',*,*,#5748,.F.);
#7371=ORIENTED_EDGE('',*,*,#5807,.T.);
#7372=ORIENTED_EDGE('',*,*,#5770,.T.);
#7373=ORIENTED_EDGE('',*,*,#5814,.F.);
#7374=ORIENTED_EDGE('',*,*,#5750,.F.);
#7375=ORIENTED_EDGE('',*,*,#5813,.T.);
#7376=ORIENTED_EDGE('',*,*,#5720,.F.);
#7377=ORIENTED_EDGE('',*,*,#5723,.F.);
#7378=ORIENTED_EDGE('',*,*,#5726,.F.);
#7379=ORIENTED_EDGE('',*,*,#5729,.F.);
#7380=ORIENTED_EDGE('',*,*,#5732,.F.);
#7381=ORIENTED_EDGE('',*,*,#5735,.F.);
#7382=ORIENTED_EDGE('',*,*,#5738,.F.);
#7383=ORIENTED_EDGE('',*,*,#5741,.F.);
#7384=ORIENTED_EDGE('',*,*,#5744,.F.);
#7385=ORIENTED_EDGE('',*,*,#5768,.T.);
#7386=ORIENTED_EDGE('',*,*,#5773,.F.);
#7387=ORIENTED_EDGE('',*,*,#5761,.F.);
#7388=ORIENTED_EDGE('',*,*,#5814,.T.);
#7389=ORIENTED_EDGE('',*,*,#5801,.F.);
#7390=ORIENTED_EDGE('',*,*,#5815,.T.);
#7391=ORIENTED_EDGE('',*,*,#5808,.T.);
#7392=ORIENTED_EDGE('',*,*,#5747,.T.);
#7393=ORIENTED_EDGE('',*,*,#5789,.T.);
#7394=ORIENTED_EDGE('',*,*,#5816,.T.);
#7395=ORIENTED_EDGE('',*,*,#5774,.F.);
#7396=ORIENTED_EDGE('',*,*,#5767,.T.);
#7397=ORIENTED_EDGE('',*,*,#5787,.F.);
#7398=ORIENTED_EDGE('',*,*,#5817,.T.);
#7399=ORIENTED_EDGE('',*,*,#5776,.F.);
#7400=ORIENTED_EDGE('',*,*,#5818,.T.);
#7401=ORIENTED_EDGE('',*,*,#5795,.F.);
#7402=ORIENTED_EDGE('',*,*,#5819,.T.);
#7403=ORIENTED_EDGE('',*,*,#5805,.F.);
#7404=ORIENTED_EDGE('',*,*,#5820,.T.);
#7405=ORIENTED_EDGE('',*,*,#5784,.F.);
#7406=ORIENTED_EDGE('',*,*,#5821,.T.);
#7407=ORIENTED_EDGE('',*,*,#5771,.F.);
#7408=ORIENTED_EDGE('',*,*,#5822,.T.);
#7409=ORIENTED_EDGE('',*,*,#5810,.F.);
#7410=ORIENTED_EDGE('',*,*,#5823,.T.);
#7411=ORIENTED_EDGE('',*,*,#5799,.F.);
#7412=ORIENTED_EDGE('',*,*,#5824,.T.);
#7413=ORIENTED_EDGE('',*,*,#5772,.F.);
#7414=ORIENTED_EDGE('',*,*,#5821,.F.);
#7415=ORIENTED_EDGE('',*,*,#5783,.F.);
#7416=ORIENTED_EDGE('',*,*,#5763,.F.);
#7417=ORIENTED_EDGE('',*,*,#5785,.F.);
#7418=ORIENTED_EDGE('',*,*,#5822,.F.);
#7419=ORIENTED_EDGE('',*,*,#5779,.F.);
#7420=ORIENTED_EDGE('',*,*,#5781,.F.);
#7421=ORIENTED_EDGE('',*,*,#5777,.F.);
#7422=ORIENTED_EDGE('',*,*,#5817,.F.);
#7423=ORIENTED_EDGE('',*,*,#5786,.F.);
#7424=ORIENTED_EDGE('',*,*,#5782,.F.);
#7425=ORIENTED_EDGE('',*,*,#5788,.F.);
#7426=ORIENTED_EDGE('',*,*,#5818,.F.);
#7427=ORIENTED_EDGE('',*,*,#5775,.F.);
#7428=ORIENTED_EDGE('',*,*,#5816,.F.);
#7429=ORIENTED_EDGE('',*,*,#5806,.F.);
#7430=ORIENTED_EDGE('',*,*,#5819,.F.);
#7431=ORIENTED_EDGE('',*,*,#5794,.F.);
#7432=ORIENTED_EDGE('',*,*,#5757,.F.);
#7433=ORIENTED_EDGE('',*,*,#5796,.F.);
#7434=ORIENTED_EDGE('',*,*,#5820,.F.);
#7435=ORIENTED_EDGE('',*,*,#5812,.F.);
#7436=ORIENTED_EDGE('',*,*,#5802,.F.);
#7437=ORIENTED_EDGE('',*,*,#5800,.F.);
#7438=ORIENTED_EDGE('',*,*,#5823,.F.);
#7439=ORIENTED_EDGE('',*,*,#5809,.F.);
#7440=ORIENTED_EDGE('',*,*,#5815,.F.);
#7441=ORIENTED_EDGE('',*,*,#5811,.F.);
#7442=ORIENTED_EDGE('',*,*,#5824,.F.);
#7443=ORIENTED_EDGE('',*,*,#5798,.F.);
#7444=ORIENTED_EDGE('',*,*,#5804,.F.);
#10145=CYLINDRICAL_SURFACE('',#11106,1.25);
#10146=CYLINDRICAL_SURFACE('',#11109,1.25);
#10147=CYLINDRICAL_SURFACE('',#11112,1.25);
#10148=CYLINDRICAL_SURFACE('',#11115,1.25);
#10149=CYLINDRICAL_SURFACE('',#11118,1.25);
#10150=CYLINDRICAL_SURFACE('',#11121,1.25);
#10151=CYLINDRICAL_SURFACE('',#11124,1.25);
#10152=CYLINDRICAL_SURFACE('',#11127,1.25);
#10153=CYLINDRICAL_SURFACE('',#11130,1.25);
#10154=CYLINDRICAL_SURFACE('',#11133,1.25);
#10155=CYLINDRICAL_SURFACE('',#11136,1.25);
#10156=CYLINDRICAL_SURFACE('',#11139,1.25);
#10157=CYLINDRICAL_SURFACE('',#11142,1.25);
#10158=CYLINDRICAL_SURFACE('',#11145,1.25);
#10159=CYLINDRICAL_SURFACE('',#11148,1.25);
#10160=CYLINDRICAL_SURFACE('',#11151,1.25);
#10161=CYLINDRICAL_SURFACE('',#11154,5.);
#10162=CYLINDRICAL_SURFACE('',#11184,3.);
#10163=CYLINDRICAL_SURFACE('',#11186,3.);
#10164=CYLINDRICAL_SURFACE('',#11198,6.);
#10165=CYLINDRICAL_SURFACE('',#11200,6.);
#10166=CYLINDRICAL_SURFACE('',#11207,2.5);
#10167=CYLINDRICAL_SURFACE('',#11208,2.5);
#10168=CYLINDRICAL_SURFACE('',#11209,2.5);
#10169=CYLINDRICAL_SURFACE('',#11210,2.5);
#10170=CYLINDRICAL_SURFACE('',#11211,2.5);
#10171=CYLINDRICAL_SURFACE('',#11212,2.5);
#10172=CYLINDRICAL_SURFACE('',#11213,2.5);
#10173=CYLINDRICAL_SURFACE('',#11214,2.5);
#10352=ADVANCED_FACE('',(#900),#10145,.F.);
#10353=ADVANCED_FACE('',(#901),#10146,.F.);
#10354=ADVANCED_FACE('',(#902),#10147,.F.);
#10355=ADVANCED_FACE('',(#903),#10148,.F.);
#10356=ADVANCED_FACE('',(#904),#10149,.F.);
#10357=ADVANCED_FACE('',(#905),#10150,.F.);
#10358=ADVANCED_FACE('',(#906),#10151,.F.);
#10359=ADVANCED_FACE('',(#907),#10152,.F.);
#10360=ADVANCED_FACE('',(#908),#10153,.F.);
#10361=ADVANCED_FACE('',(#909),#10154,.F.);
#10362=ADVANCED_FACE('',(#910),#10155,.F.);
#10363=ADVANCED_FACE('',(#911),#10156,.F.);
#10364=ADVANCED_FACE('',(#912),#10157,.F.);
#10365=ADVANCED_FACE('',(#913),#10158,.F.);
#10366=ADVANCED_FACE('',(#914),#10159,.F.);
#10367=ADVANCED_FACE('',(#915),#10160,.F.);
#10368=ADVANCED_FACE('',(#916),#10161,.F.);
#10369=ADVANCED_FACE('',(#917),#576,.T.);
#10370=ADVANCED_FACE('',(#918),#577,.T.);
#10371=ADVANCED_FACE('',(#919),#578,.T.);
#10372=ADVANCED_FACE('',(#920),#579,.T.);
#10373=ADVANCED_FACE('',(#921),#580,.T.);
#10374=ADVANCED_FACE('',(#922),#581,.T.);
#10375=ADVANCED_FACE('',(#923),#582,.T.);
#10376=ADVANCED_FACE('',(#924),#583,.T.);
#10377=ADVANCED_FACE('',(#925,#380,#381,#382,#383),#584,.F.);
#10378=ADVANCED_FACE('',(#926),#585,.T.);
#10379=ADVANCED_FACE('',(#927,#384,#385,#386,#387),#586,.T.);
#10380=ADVANCED_FACE('',(#928),#10162,.F.);
#10381=ADVANCED_FACE('',(#929,#388,#389,#390,#391,#392,#393,#394,#395,#396),
#587,.T.);
#10382=ADVANCED_FACE('',(#930),#10163,.F.);
#10383=ADVANCED_FACE('',(#931,#397,#398,#399,#400),#588,.T.);
#10384=ADVANCED_FACE('',(#932),#589,.T.);
#10385=ADVANCED_FACE('',(#933,#401,#402,#403,#404),#590,.F.);
#10386=ADVANCED_FACE('',(#934),#10164,.T.);
#10387=ADVANCED_FACE('',(#935,#405,#406,#407,#408,#409,#410,#411,#412,#413),
#591,.F.);
#10388=ADVANCED_FACE('',(#936),#10165,.T.);
#10389=ADVANCED_FACE('',(#937),#592,.F.);
#10390=ADVANCED_FACE('',(#938),#593,.T.);
#10391=ADVANCED_FACE('',(#939),#594,.F.);
#10392=ADVANCED_FACE('',(#940),#595,.F.);
#10393=ADVANCED_FACE('',(#941),#596,.F.);
#10394=ADVANCED_FACE('',(#942),#597,.T.);
#10395=ADVANCED_FACE('',(#943),#10166,.T.);
#10396=ADVANCED_FACE('',(#944),#10167,.T.);
#10397=ADVANCED_FACE('',(#945),#10168,.T.);
#10398=ADVANCED_FACE('',(#946),#10169,.T.);
#10399=ADVANCED_FACE('',(#947),#10170,.T.);
#10400=ADVANCED_FACE('',(#948),#10171,.T.);
#10401=ADVANCED_FACE('',(#949),#10172,.T.);
#10402=ADVANCED_FACE('',(#950),#10173,.T.);
#10944=CLOSED_SHELL('',(#10352,#10353,#10354,#10355,#10356,#10357,#10358,
#10359,#10360,#10361,#10362,#10363,#10364,#10365,#10366,#10367,#10368,#10369,
#10370,#10371,#10372,#10373,#10374,#10375,#10376,#10377,#10378,#10379,#10380,
#10381,#10382,#10383,#10384,#10385,#10386,#10387,#10388,#10389,#10390,#10391,
#10392,#10393,#10394,#10395,#10396,#10397,#10398,#10399,#10400,#10401,#10402));
#11105=AXIS2_PLACEMENT_3D('',#15423,#12216,#12217);
#11106=AXIS2_PLACEMENT_3D('',#15424,#12218,#12219);
#11107=AXIS2_PLACEMENT_3D('',#15426,#12220,#12221);
#11108=AXIS2_PLACEMENT_3D('',#15429,#12223,#12224);
#11109=AXIS2_PLACEMENT_3D('',#15430,#12225,#12226);
#11110=AXIS2_PLACEMENT_3D('',#15432,#12227,#12228);
#11111=AXIS2_PLACEMENT_3D('',#15435,#12230,#12231);
#11112=AXIS2_PLACEMENT_3D('',#15436,#12232,#12233);
#11113=AXIS2_PLACEMENT_3D('',#15438,#12234,#12235);
#11114=AXIS2_PLACEMENT_3D('',#15441,#12237,#12238);
#11115=AXIS2_PLACEMENT_3D('',#15442,#12239,#12240);
#11116=AXIS2_PLACEMENT_3D('',#15444,#12241,#12242);
#11117=AXIS2_PLACEMENT_3D('',#15447,#12244,#12245);
#11118=AXIS2_PLACEMENT_3D('',#15448,#12246,#12247);
#11119=AXIS2_PLACEMENT_3D('',#15450,#12248,#12249);
#11120=AXIS2_PLACEMENT_3D('',#15453,#12251,#12252);
#11121=AXIS2_PLACEMENT_3D('',#15454,#12253,#12254);
#11122=AXIS2_PLACEMENT_3D('',#15456,#12255,#12256);
#11123=AXIS2_PLACEMENT_3D('',#15459,#12258,#12259);
#11124=AXIS2_PLACEMENT_3D('',#15460,#12260,#12261);
#11125=AXIS2_PLACEMENT_3D('',#15462,#12262,#12263);
#11126=AXIS2_PLACEMENT_3D('',#15465,#12265,#12266);
#11127=AXIS2_PLACEMENT_3D('',#15466,#12267,#12268);
#11128=AXIS2_PLACEMENT_3D('',#15468,#12269,#12270);
#11129=AXIS2_PLACEMENT_3D('',#15471,#12272,#12273);
#11130=AXIS2_PLACEMENT_3D('',#15472,#12274,#12275);
#11131=AXIS2_PLACEMENT_3D('',#15474,#12276,#12277);
#11132=AXIS2_PLACEMENT_3D('',#15477,#12279,#12280);
#11133=AXIS2_PLACEMENT_3D('',#15478,#12281,#12282);
#11134=AXIS2_PLACEMENT_3D('',#15480,#12283,#12284);
#11135=AXIS2_PLACEMENT_3D('',#15483,#12286,#12287);
#11136=AXIS2_PLACEMENT_3D('',#15484,#12288,#12289);
#11137=AXIS2_PLACEMENT_3D('',#15486,#12290,#12291);
#11138=AXIS2_PLACEMENT_3D('',#15489,#12293,#12294);
#11139=AXIS2_PLACEMENT_3D('',#15490,#12295,#12296);
#11140=AXIS2_PLACEMENT_3D('',#15492,#12297,#12298);
#11141=AXIS2_PLACEMENT_3D('',#15495,#12300,#12301);
#11142=AXIS2_PLACEMENT_3D('',#15496,#12302,#12303);
#11143=AXIS2_PLACEMENT_3D('',#15498,#12304,#12305);
#11144=AXIS2_PLACEMENT_3D('',#15501,#12307,#12308);
#11145=AXIS2_PLACEMENT_3D('',#15502,#12309,#12310);
#11146=AXIS2_PLACEMENT_3D('',#15504,#12311,#12312);
#11147=AXIS2_PLACEMENT_3D('',#15507,#12314,#12315);
#11148=AXIS2_PLACEMENT_3D('',#15508,#12316,#12317);
#11149=AXIS2_PLACEMENT_3D('',#15510,#12318,#12319);
#11150=AXIS2_PLACEMENT_3D('',#15513,#12321,#12322);
#11151=AXIS2_PLACEMENT_3D('',#15514,#12323,#12324);
#11152=AXIS2_PLACEMENT_3D('',#15516,#12325,#12326);
#11153=AXIS2_PLACEMENT_3D('',#15519,#12328,#12329);
#11154=AXIS2_PLACEMENT_3D('',#15520,#12330,#12331);
#11155=AXIS2_PLACEMENT_3D('',#15522,#12332,#12333);
#11156=AXIS2_PLACEMENT_3D('',#15525,#12335,#12336);
#11157=AXIS2_PLACEMENT_3D('',#15526,#12337,#12338);
#11158=AXIS2_PLACEMENT_3D('',#15531,#12340,#12341);
#11159=AXIS2_PLACEMENT_3D('',#15534,#12343,#12344);
#11160=AXIS2_PLACEMENT_3D('',#15535,#12345,#12346);
#11161=AXIS2_PLACEMENT_3D('',#15541,#12350,#12351);
#11162=AXIS2_PLACEMENT_3D('',#15546,#12353,#12354);
#11163=AXIS2_PLACEMENT_3D('',#15549,#12356,#12357);
#11164=AXIS2_PLACEMENT_3D('',#15550,#12358,#12359);
#11165=AXIS2_PLACEMENT_3D('',#15556,#12363,#12364);
#11166=AXIS2_PLACEMENT_3D('',#15560,#12366,#12367);
#11167=AXIS2_PLACEMENT_3D('',#15561,#12368,#12369);
#11168=AXIS2_PLACEMENT_3D('',#15562,#12370,#12371);
#11169=AXIS2_PLACEMENT_3D('',#15568,#12375,#12376);
#11170=AXIS2_PLACEMENT_3D('',#15573,#12378,#12379);
#11171=AXIS2_PLACEMENT_3D('',#15576,#12381,#12382);
#11172=AXIS2_PLACEMENT_3D('',#15577,#12383,#12384);
#11173=AXIS2_PLACEMENT_3D('',#15580,#12387,#12388);
#11174=AXIS2_PLACEMENT_3D('',#15584,#12390,#12391);
#11175=AXIS2_PLACEMENT_3D('',#15589,#12394,#12395);
#11176=AXIS2_PLACEMENT_3D('',#15593,#12397,#12398);
#11177=AXIS2_PLACEMENT_3D('',#15596,#12400,#12401);
#11178=AXIS2_PLACEMENT_3D('',#15597,#12402,#12403);
#11179=AXIS2_PLACEMENT_3D('',#15603,#12407,#12408);
#11180=AXIS2_PLACEMENT_3D('',#15605,#12409,#12410);
#11181=AXIS2_PLACEMENT_3D('',#15608,#12412,#12413);
#11182=AXIS2_PLACEMENT_3D('',#15610,#12414,#12415);
#11183=AXIS2_PLACEMENT_3D('',#15614,#12417,#12418);
#11184=AXIS2_PLACEMENT_3D('',#15617,#12421,#12422);
#11185=AXIS2_PLACEMENT_3D('',#15619,#12424,#12425);
#11186=AXIS2_PLACEMENT_3D('',#15621,#12427,#12428);
#11187=AXIS2_PLACEMENT_3D('',#15623,#12430,#12431);
#11188=AXIS2_PLACEMENT_3D('',#15625,#12432,#12433);
#11189=AXIS2_PLACEMENT_3D('',#15629,#12435,#12436);
#11190=AXIS2_PLACEMENT_3D('',#15633,#12438,#12439);
#11191=AXIS2_PLACEMENT_3D('',#15637,#12441,#12442);
#11192=AXIS2_PLACEMENT_3D('',#15639,#12444,#12445);
#11193=AXIS2_PLACEMENT_3D('',#15645,#12449,#12450);
#11194=AXIS2_PLACEMENT_3D('',#15649,#12452,#12453);
#11195=AXIS2_PLACEMENT_3D('',#15654,#12456,#12457);
#11196=AXIS2_PLACEMENT_3D('',#15657,#12459,#12460);
#11197=AXIS2_PLACEMENT_3D('',#15658,#12461,#12462);
#11198=AXIS2_PLACEMENT_3D('',#15659,#12463,#12464);
#11199=AXIS2_PLACEMENT_3D('',#15661,#12466,#12467);
#11200=AXIS2_PLACEMENT_3D('',#15663,#12469,#12470);
#11201=AXIS2_PLACEMENT_3D('',#15664,#12471,#12472);
#11202=AXIS2_PLACEMENT_3D('',#15666,#12474,#12475);
#11203=AXIS2_PLACEMENT_3D('',#15668,#12477,#12478);
#11204=AXIS2_PLACEMENT_3D('',#15671,#12481,#12482);
#11205=AXIS2_PLACEMENT_3D('',#15674,#12485,#12486);
#11206=AXIS2_PLACEMENT_3D('',#15677,#12489,#12490);
#11207=AXIS2_PLACEMENT_3D('',#15680,#12493,#12494);
#11208=AXIS2_PLACEMENT_3D('',#15681,#12495,#12496);
#11209=AXIS2_PLACEMENT_3D('',#15682,#12497,#12498);
#11210=AXIS2_PLACEMENT_3D('',#15683,#12499,#12500);
#11211=AXIS2_PLACEMENT_3D('',#15684,#12501,#12502);
#11212=AXIS2_PLACEMENT_3D('',#15685,#12503,#12504);
#11213=AXIS2_PLACEMENT_3D('',#15686,#12505,#12506);
#11214=AXIS2_PLACEMENT_3D('',#15687,#12507,#12508);
#12216=DIRECTION('axis',(0.,0.,1.));
#12217=DIRECTION('refdir',(1.,0.,0.));
#12218=DIRECTION('center_axis',(0.,1.,0.));
#12219=DIRECTION('ref_axis',(0.,0.,1.));
#12220=DIRECTION('center_axis',(0.,1.,0.));
#12221=DIRECTION('ref_axis',(0.,0.,-1.));
#12222=DIRECTION('',(0.,1.,0.));
#12223=DIRECTION('center_axis',(0.,1.,0.));
#12224=DIRECTION('ref_axis',(0.,0.,1.));
#12225=DIRECTION('center_axis',(0.,1.,0.));
#12226=DIRECTION('ref_axis',(0.,0.,1.));
#12227=DIRECTION('center_axis',(0.,-1.,0.));
#12228=DIRECTION('ref_axis',(0.,0.,-1.));
#12229=DIRECTION('',(0.,1.,0.));
#12230=DIRECTION('center_axis',(0.,1.,0.));
#12231=DIRECTION('ref_axis',(0.,0.,-1.));
#12232=DIRECTION('center_axis',(0.,1.,0.));
#12233=DIRECTION('ref_axis',(0.,0.,1.));
#12234=DIRECTION('center_axis',(0.,1.,0.));
#12235=DIRECTION('ref_axis',(0.,0.,-1.));
#12236=DIRECTION('',(0.,1.,0.));
#12237=DIRECTION('center_axis',(0.,1.,0.));
#12238=DIRECTION('ref_axis',(0.,0.,1.));
#12239=DIRECTION('center_axis',(0.,1.,0.));
#12240=DIRECTION('ref_axis',(0.,0.,1.));
#12241=DIRECTION('center_axis',(0.,-1.,0.));
#12242=DIRECTION('ref_axis',(0.,0.,-1.));
#12243=DIRECTION('',(0.,1.,0.));
#12244=DIRECTION('center_axis',(0.,1.,0.));
#12245=DIRECTION('ref_axis',(0.,0.,-1.));
#12246=DIRECTION('center_axis',(0.,1.,0.));
#12247=DIRECTION('ref_axis',(0.,0.,1.));
#12248=DIRECTION('center_axis',(0.,1.,0.));
#12249=DIRECTION('ref_axis',(0.,0.,1.));
#12250=DIRECTION('',(0.,1.,0.));
#12251=DIRECTION('center_axis',(0.,1.,0.));
#12252=DIRECTION('ref_axis',(0.,0.,1.));
#12253=DIRECTION('center_axis',(0.,1.,0.));
#12254=DIRECTION('ref_axis',(0.,0.,1.));
#12255=DIRECTION('center_axis',(0.,-1.,0.));
#12256=DIRECTION('ref_axis',(0.,0.,-1.));
#12257=DIRECTION('',(0.,1.,0.));
#12258=DIRECTION('center_axis',(0.,1.,0.));
#12259=DIRECTION('ref_axis',(0.,0.,1.));
#12260=DIRECTION('center_axis',(0.,1.,0.));
#12261=DIRECTION('ref_axis',(0.,0.,1.));
#12262=DIRECTION('center_axis',(0.,1.,0.));
#12263=DIRECTION('ref_axis',(0.,0.,1.));
#12264=DIRECTION('',(0.,1.,0.));
#12265=DIRECTION('center_axis',(0.,1.,0.));
#12266=DIRECTION('ref_axis',(0.,0.,1.));
#12267=DIRECTION('center_axis',(0.,1.,0.));
#12268=DIRECTION('ref_axis',(0.,0.,1.));
#12269=DIRECTION('center_axis',(0.,-1.,0.));
#12270=DIRECTION('ref_axis',(0.,0.,-1.));
#12271=DIRECTION('',(0.,1.,0.));
#12272=DIRECTION('center_axis',(0.,1.,0.));
#12273=DIRECTION('ref_axis',(0.,0.,1.));
#12274=DIRECTION('center_axis',(-1.,-3.22196856956734E-16,0.));
#12275=DIRECTION('ref_axis',(3.22196856956734E-16,-1.,0.));
#12276=DIRECTION('center_axis',(1.,0.,0.));
#12277=DIRECTION('ref_axis',(0.,0.,-1.));
#12278=DIRECTION('',(-1.,-3.22196856956734E-16,0.));
#12279=DIRECTION('center_axis',(-1.,-3.22196856956734E-16,0.));
#12280=DIRECTION('ref_axis',(3.22196856956734E-16,-1.,0.));
#12281=DIRECTION('center_axis',(-1.,-3.22196856956734E-16,0.));
#12282=DIRECTION('ref_axis',(3.22196856956734E-16,-1.,0.));
#12283=DIRECTION('center_axis',(1.,0.,0.));
#12284=DIRECTION('ref_axis',(0.,0.,-1.));
#12285=DIRECTION('',(-1.,-3.22196856956734E-16,0.));
#12286=DIRECTION('center_axis',(-1.,-3.22196856956734E-16,0.));
#12287=DIRECTION('ref_axis',(3.22196856956734E-16,-1.,0.));
#12288=DIRECTION('center_axis',(-1.,-3.22196856956734E-16,0.));
#12289=DIRECTION('ref_axis',(3.22196856956734E-16,-1.,0.));
#12290=DIRECTION('center_axis',(1.,0.,0.));
#12291=DIRECTION('ref_axis',(0.,0.,-1.));
#12292=DIRECTION('',(-1.,-3.22196856956734E-16,0.));
#12293=DIRECTION('center_axis',(-1.,-3.22196856956734E-16,0.));
#12294=DIRECTION('ref_axis',(3.22196856956734E-16,-1.,0.));
#12295=DIRECTION('center_axis',(-1.,-3.22196856956734E-16,0.));
#12296=DIRECTION('ref_axis',(3.22196856956734E-16,-1.,0.));
#12297=DIRECTION('center_axis',(1.,0.,0.));
#12298=DIRECTION('ref_axis',(0.,0.,-1.));
#12299=DIRECTION('',(-1.,-3.22196856956734E-16,0.));
#12300=DIRECTION('center_axis',(-1.,-3.22196856956734E-16,0.));
#12301=DIRECTION('ref_axis',(3.22196856956734E-16,-1.,0.));
#12302=DIRECTION('center_axis',(-1.,-3.22196856956734E-16,0.));
#12303=DIRECTION('ref_axis',(3.22196856956734E-16,-1.,0.));
#12304=DIRECTION('center_axis',(1.,0.,0.));
#12305=DIRECTION('ref_axis',(0.,0.,-1.));
#12306=DIRECTION('',(-1.,-3.22196856956734E-16,0.));
#12307=DIRECTION('center_axis',(-1.,-3.22196856956734E-16,0.));
#12308=DIRECTION('ref_axis',(3.22196856956734E-16,-1.,0.));
#12309=DIRECTION('center_axis',(-1.,-3.22196856956734E-16,0.));
#12310=DIRECTION('ref_axis',(3.22196856956734E-16,-1.,0.));
#12311=DIRECTION('center_axis',(1.,0.,0.));
#12312=DIRECTION('ref_axis',(0.,0.,-1.));
#12313=DIRECTION('',(-1.,-3.22196856956734E-16,0.));
#12314=DIRECTION('center_axis',(-1.,-3.22196856956734E-16,0.));
#12315=DIRECTION('ref_axis',(3.22196856956734E-16,-1.,0.));
#12316=DIRECTION('center_axis',(-1.,-3.22196856956734E-16,0.));
#12317=DIRECTION('ref_axis',(3.22196856956734E-16,-1.,0.));
#12318=DIRECTION('center_axis',(1.,0.,0.));
#12319=DIRECTION('ref_axis',(0.,0.,-1.));
#12320=DIRECTION('',(-1.,-3.22196856956734E-16,0.));
#12321=DIRECTION('center_axis',(-1.,-3.22196856956734E-16,0.));
#12322=DIRECTION('ref_axis',(3.22196856956734E-16,-1.,0.));
#12323=DIRECTION('center_axis',(-1.,-3.22196856956734E-16,0.));
#12324=DIRECTION('ref_axis',(3.22196856956734E-16,-1.,0.));
#12325=DIRECTION('center_axis',(1.,0.,0.));
#12326=DIRECTION('ref_axis',(0.,0.,-1.));
#12327=DIRECTION('',(-1.,-3.22196856956734E-16,0.));
#12328=DIRECTION('center_axis',(-1.,-3.22196856956734E-16,0.));
#12329=DIRECTION('ref_axis',(3.22196856956734E-16,-1.,0.));
#12330=DIRECTION('center_axis',(-1.,-3.22196856956734E-16,0.));
#12331=DIRECTION('ref_axis',(3.22196856956734E-16,-1.,0.));
#12332=DIRECTION('center_axis',(1.,0.,0.));
#12333=DIRECTION('ref_axis',(0.,0.,-1.));
#12334=DIRECTION('',(-1.,-3.22196856956734E-16,0.));
#12335=DIRECTION('center_axis',(-1.,-3.22196856956734E-16,0.));
#12336=DIRECTION('ref_axis',(3.22196856956734E-16,-1.,0.));
#12337=DIRECTION('center_axis',(0.,0.,1.));
#12338=DIRECTION('ref_axis',(1.,0.,0.));
#12339=DIRECTION('',(-1.,0.,0.));
#12340=DIRECTION('center_axis',(0.,0.,1.));
#12341=DIRECTION('ref_axis',(-1.,0.,0.));
#12342=DIRECTION('',(-1.44560289664734E-16,-1.,0.));
#12343=DIRECTION('center_axis',(0.,0.,1.));
#12344=DIRECTION('ref_axis',(1.,0.,0.));
#12345=DIRECTION('center_axis',(0.,0.,1.));
#12346=DIRECTION('ref_axis',(1.,0.,0.));
#12347=DIRECTION('',(3.22196856956734E-16,-1.,0.));
#12348=DIRECTION('',(0.,-1.,0.));
#12349=DIRECTION('',(1.,0.,0.));
#12350=DIRECTION('center_axis',(0.,0.,-1.));
#12351=DIRECTION('ref_axis',(-1.,0.,0.));
#12352=DIRECTION('',(1.44560289664734E-16,1.,0.));
#12353=DIRECTION('center_axis',(0.,0.,1.));
#12354=DIRECTION('ref_axis',(-1.,0.,0.));
#12355=DIRECTION('',(1.,0.,0.));
#12356=DIRECTION('center_axis',(0.,0.,1.));
#12357=DIRECTION('ref_axis',(1.,0.,0.));
#12358=DIRECTION('center_axis',(0.,0.,-1.));
#12359=DIRECTION('ref_axis',(-1.,0.,0.));
#12360=DIRECTION('',(-1.,0.,0.));
#12361=DIRECTION('',(0.,-1.,0.));
#12362=DIRECTION('',(-1.,0.,0.));
#12363=DIRECTION('center_axis',(0.,0.,1.));
#12364=DIRECTION('ref_axis',(1.,0.,0.));
#12365=DIRECTION('',(0.,-1.,0.));
#12366=DIRECTION('center_axis',(0.,0.,1.));
#12367=DIRECTION('ref_axis',(-1.,-1.15648231731787E-15,0.));
#12368=DIRECTION('center_axis',(0.,0.,1.));
#12369=DIRECTION('ref_axis',(1.,0.,0.));
#12370=DIRECTION('center_axis',(0.,0.,1.));
#12371=DIRECTION('ref_axis',(1.,0.,0.));
#12372=DIRECTION('',(1.,0.,0.));
#12373=DIRECTION('',(0.,1.,0.));
#12374=DIRECTION('',(1.,0.,0.));
#12375=DIRECTION('center_axis',(0.,0.,-1.));
#12376=DIRECTION('ref_axis',(-1.,0.,0.));
#12377=DIRECTION('',(-1.,0.,0.));
#12378=DIRECTION('center_axis',(0.,0.,1.));
#12379=DIRECTION('ref_axis',(-1.,-1.15648231731787E-15,0.));
#12380=DIRECTION('',(0.,1.,0.));
#12381=DIRECTION('center_axis',(0.,0.,1.));
#12382=DIRECTION('ref_axis',(1.,0.,0.));
#12383=DIRECTION('center_axis',(0.,0.,-1.));
#12384=DIRECTION('ref_axis',(-1.,0.,0.));
#12385=DIRECTION('',(0.,-1.,0.));
#12386=DIRECTION('',(3.22196856956734E-16,-1.,0.));
#12387=DIRECTION('center_axis',(0.,1.,0.));
#12388=DIRECTION('ref_axis',(0.,0.,1.));
#12389=DIRECTION('',(-0.707106781186549,0.,0.707106781186547));
#12390=DIRECTION('center_axis',(0.,-1.,0.));
#12391=DIRECTION('ref_axis',(5.20417042793042E-15,0.,1.));
#12392=DIRECTION('',(0.,0.,-1.));
#12393=DIRECTION('',(1.,0.,0.));
#12394=DIRECTION('center_axis',(0.,-1.,0.));
#12395=DIRECTION('ref_axis',(0.,0.,1.));
#12396=DIRECTION('',(0.707106781186546,0.,0.707106781186549));
#12397=DIRECTION('center_axis',(0.,-1.,0.));
#12398=DIRECTION('ref_axis',(0.,0.,1.));
#12399=DIRECTION('',(0.,0.,-1.));
#12400=DIRECTION('center_axis',(0.,-1.,0.));
#12401=DIRECTION('ref_axis',(-1.31838984174237E-14,0.,1.));
#12402=DIRECTION('center_axis',(1.,0.,0.));
#12403=DIRECTION('ref_axis',(0.,0.,-1.));
#12404=DIRECTION('',(0.,0.,-1.));
#12405=DIRECTION('',(0.,-1.,0.));
#12406=DIRECTION('',(0.,1.,0.));
#12407=DIRECTION('center_axis',(0.,1.,0.));
#12408=DIRECTION('ref_axis',(0.,0.,1.));
#12409=DIRECTION('center_axis',(0.,1.,0.));
#12410=DIRECTION('ref_axis',(0.,0.,1.));
#12411=DIRECTION('',(0.707106781186549,0.,-0.707106781186547));
#12412=DIRECTION('center_axis',(0.,1.,0.));
#12413=DIRECTION('ref_axis',(0.,0.,1.));
#12414=DIRECTION('center_axis',(0.,1.,0.));
#12415=DIRECTION('ref_axis',(0.,0.,1.));
#12416=DIRECTION('',(-0.707106781186546,0.,-0.707106781186549));
#12417=DIRECTION('center_axis',(0.,1.,0.));
#12418=DIRECTION('ref_axis',(0.,0.,1.));
#12419=DIRECTION('',(1.,0.,0.));
#12420=DIRECTION('',(0.,0.,-1.));
#12421=DIRECTION('center_axis',(0.,0.,-1.));
#12422=DIRECTION('ref_axis',(-1.,0.,0.));
#12423=DIRECTION('',(0.,0.,-1.));
#12424=DIRECTION('center_axis',(1.,0.,0.));
#12425=DIRECTION('ref_axis',(0.,0.,-1.));
#12426=DIRECTION('',(0.,0.,-1.));
#12427=DIRECTION('center_axis',(0.,0.,-1.));
#12428=DIRECTION('ref_axis',(-1.,0.,0.));
#12429=DIRECTION('',(0.,0.,-1.));
#12430=DIRECTION('center_axis',(0.,-1.,0.));
#12431=DIRECTION('ref_axis',(0.,0.,-1.));
#12432=DIRECTION('center_axis',(0.,-1.,0.));
#12433=DIRECTION('ref_axis',(0.,0.,-1.));
#12434=DIRECTION('',(0.707106781186545,0.,0.70710678118655));
#12435=DIRECTION('center_axis',(0.,-1.,0.));
#12436=DIRECTION('ref_axis',(0.,0.,-1.));
#12437=DIRECTION('',(0.,0.,-1.));
#12438=DIRECTION('center_axis',(0.,-1.,0.));
#12439=DIRECTION('ref_axis',(0.,0.,-1.));
#12440=DIRECTION('',(-0.707106781186549,0.,0.707106781186547));
#12441=DIRECTION('center_axis',(0.,-1.,0.));
#12442=DIRECTION('ref_axis',(0.,0.,-1.));
#12443=DIRECTION('',(-1.,0.,0.));
#12444=DIRECTION('center_axis',(1.,0.,0.));
#12445=DIRECTION('ref_axis',(0.,0.,-1.));
#12446=DIRECTION('',(0.,1.,0.));
#12447=DIRECTION('',(0.,0.,-1.));
#12448=DIRECTION('',(0.,-1.,0.));
#12449=DIRECTION('center_axis',(0.,-1.,0.));
#12450=DIRECTION('ref_axis',(0.,0.,-1.));
#12451=DIRECTION('',(-0.707106781186545,0.,-0.70710678118655));
#12452=DIRECTION('center_axis',(0.,1.,0.));
#12453=DIRECTION('ref_axis',(1.04083408558608E-15,0.,-1.));
#12454=DIRECTION('',(0.,0.,-1.));
#12455=DIRECTION('',(-1.,0.,0.));
#12456=DIRECTION('center_axis',(0.,1.,0.));
#12457=DIRECTION('ref_axis',(5.20417042793042E-15,0.,-1.));
#12458=DIRECTION('',(0.707106781186549,0.,-0.707106781186546));
#12459=DIRECTION('center_axis',(0.,1.,0.));
#12460=DIRECTION('ref_axis',(-1.59594559789866E-14,0.,-1.));
#12461=DIRECTION('center_axis',(0.,1.,0.));
#12462=DIRECTION('ref_axis',(2.77555756156289E-15,0.,-1.));
#12463=DIRECTION('center_axis',(0.,0.,-1.));
#12464=DIRECTION('ref_axis',(-1.,0.,0.));
#12465=DIRECTION('',(0.,0.,-1.));
#12466=DIRECTION('center_axis',(1.,3.22196856956734E-16,0.));
#12467=DIRECTION('ref_axis',(-3.22196856956734E-16,1.,0.));
#12468=DIRECTION('',(0.,0.,-1.));
#12469=DIRECTION('center_axis',(0.,0.,-1.));
#12470=DIRECTION('ref_axis',(-1.,0.,0.));
#12471=DIRECTION('center_axis',(0.,0.,-1.));
#12472=DIRECTION('ref_axis',(-1.,0.,0.));
#12473=DIRECTION('',(0.,1.,0.));
#12474=DIRECTION('center_axis',(0.,0.,-1.));
#12475=DIRECTION('ref_axis',(-1.,0.,0.));
#12476=DIRECTION('',(0.,-1.,0.));
#12477=DIRECTION('center_axis',(-0.707106781186549,0.,0.707106781186546));
#12478=DIRECTION('ref_axis',(0.,-1.,0.));
#12479=DIRECTION('',(0.,-1.,0.));
#12480=DIRECTION('',(0.,1.,0.));
#12481=DIRECTION('center_axis',(-0.70710678118655,0.,0.707106781186545));
#12482=DIRECTION('ref_axis',(0.,-1.,0.));
#12483=DIRECTION('',(0.,1.,0.));
#12484=DIRECTION('',(0.,-1.,0.));
#12485=DIRECTION('center_axis',(-0.707106781186546,0.,-0.707106781186549));
#12486=DIRECTION('ref_axis',(0.,-1.,0.));
#12487=DIRECTION('',(0.,-1.,0.));
#12488=DIRECTION('',(0.,1.,0.));
#12489=DIRECTION('center_axis',(0.707106781186547,0.,0.707106781186548));
#12490=DIRECTION('ref_axis',(0.,1.,0.));
#12491=DIRECTION('',(0.,-1.,0.));
#12492=DIRECTION('',(0.,1.,0.));
#12493=DIRECTION('center_axis',(0.,-1.,0.));
#12494=DIRECTION('ref_axis',(0.,0.,-1.));
#12495=DIRECTION('center_axis',(0.,1.,0.));
#12496=DIRECTION('ref_axis',(0.,0.,1.));
#12497=DIRECTION('center_axis',(0.,-1.,0.));
#12498=DIRECTION('ref_axis',(0.,0.,-1.));
#12499=DIRECTION('center_axis',(0.,1.,0.));
#12500=DIRECTION('ref_axis',(0.,0.,1.));
#12501=DIRECTION('center_axis',(0.,1.,0.));
#12502=DIRECTION('ref_axis',(0.,0.,1.));
#12503=DIRECTION('center_axis',(0.,-1.,0.));
#12504=DIRECTION('ref_axis',(0.,0.,-1.));
#12505=DIRECTION('center_axis',(0.,-1.,0.));
#12506=DIRECTION('ref_axis',(0.,0.,-1.));
#12507=DIRECTION('center_axis',(0.,-1.,0.));
#12508=DIRECTION('ref_axis',(0.,0.,-1.));
#15423=CARTESIAN_POINT('',(0.,0.,0.));
#15424=CARTESIAN_POINT('Origin',(7.20000000000006,-20.,9.10000000000001));
#15425=CARTESIAN_POINT('',(7.20000000000006,-20.,7.85000000000001));
#15426=CARTESIAN_POINT('Origin',(7.20000000000006,-20.,9.10000000000001));
#15427=CARTESIAN_POINT('',(7.20000000000006,-17.,7.85000000000001));
#15428=CARTESIAN_POINT('',(7.20000000000006,-20.,7.85000000000001));
#15429=CARTESIAN_POINT('Origin',(7.20000000000006,-17.,9.10000000000001));
#15430=CARTESIAN_POINT('Origin',(7.20000000000006,-20.,9.10000000000001));
#15431=CARTESIAN_POINT('',(7.20000000000006,17.,7.85000000000001));
#15432=CARTESIAN_POINT('Origin',(7.20000000000006,17.,9.10000000000001));
#15433=CARTESIAN_POINT('',(7.20000000000006,20.,7.85000000000001));
#15434=CARTESIAN_POINT('',(7.20000000000006,-20.,7.85000000000001));
#15435=CARTESIAN_POINT('Origin',(7.20000000000006,20.,9.10000000000001));
#15436=CARTESIAN_POINT('Origin',(7.20000000000002,-20.,30.1));
#15437=CARTESIAN_POINT('',(7.20000000000002,-20.,28.85));
#15438=CARTESIAN_POINT('Origin',(7.20000000000002,-20.,30.1));
#15439=CARTESIAN_POINT('',(7.20000000000002,-17.,28.85));
#15440=CARTESIAN_POINT('',(7.20000000000002,-20.,28.85));
#15441=CARTESIAN_POINT('Origin',(7.20000000000002,-17.,30.1));
#15442=CARTESIAN_POINT('Origin',(7.20000000000002,-20.,30.1));
#15443=CARTESIAN_POINT('',(7.20000000000002,17.,28.85));
#15444=CARTESIAN_POINT('Origin',(7.20000000000002,17.,30.1));
#15445=CARTESIAN_POINT('',(7.20000000000002,20.,28.85));
#15446=CARTESIAN_POINT('',(7.20000000000002,-20.,28.85));
#15447=CARTESIAN_POINT('Origin',(7.20000000000002,20.,30.1));
#15448=CARTESIAN_POINT('Origin',(7.2,-20.,58.1));
#15449=CARTESIAN_POINT('',(7.2,-20.,56.85));
#15450=CARTESIAN_POINT('Origin',(7.2,-20.,58.1));
#15451=CARTESIAN_POINT('',(7.2,-17.,56.85));
#15452=CARTESIAN_POINT('',(7.2,-20.,56.85));
#15453=CARTESIAN_POINT('Origin',(7.2,-17.,58.1));
#15454=CARTESIAN_POINT('Origin',(7.2,-20.,58.1));
#15455=CARTESIAN_POINT('',(7.2,17.,56.85));
#15456=CARTESIAN_POINT('Origin',(7.2,17.,58.1));
#15457=CARTESIAN_POINT('',(7.2,20.,56.85));
#15458=CARTESIAN_POINT('',(7.2,-20.,56.85));
#15459=CARTESIAN_POINT('Origin',(7.2,20.,58.1));
#15460=CARTESIAN_POINT('Origin',(7.2,-20.,79.1));
#15461=CARTESIAN_POINT('',(7.2,-20.,77.85));
#15462=CARTESIAN_POINT('Origin',(7.2,-20.,79.1));
#15463=CARTESIAN_POINT('',(7.2,-17.,77.85));
#15464=CARTESIAN_POINT('',(7.2,-20.,77.85));
#15465=CARTESIAN_POINT('Origin',(7.2,-17.,79.1));
#15466=CARTESIAN_POINT('Origin',(7.2,-20.,79.1));
#15467=CARTESIAN_POINT('',(7.2,17.,77.85));
#15468=CARTESIAN_POINT('Origin',(7.2,17.,79.1));
#15469=CARTESIAN_POINT('',(7.2,20.,77.85));
#15470=CARTESIAN_POINT('',(7.2,-20.,77.85));
#15471=CARTESIAN_POINT('Origin',(7.2,20.,79.1));
#15472=CARTESIAN_POINT('Origin',(10.,7.77817459305203,36.321825406948));
#15473=CARTESIAN_POINT('',(0.,9.02817459305202,36.321825406948));
#15474=CARTESIAN_POINT('Origin',(0.,7.77817459305203,36.321825406948));
#15475=CARTESIAN_POINT('',(-3.,9.02817459305202,36.321825406948));
#15476=CARTESIAN_POINT('',(10.,9.02817459305203,36.321825406948));
#15477=CARTESIAN_POINT('Origin',(-3.,7.77817459305203,36.321825406948));
#15478=CARTESIAN_POINT('Origin',(10.,1.70997563773818E-14,33.1));
#15479=CARTESIAN_POINT('',(0.,1.25000000000001,33.1));
#15480=CARTESIAN_POINT('Origin',(0.,1.38777878078145E-14,33.1));
#15481=CARTESIAN_POINT('',(-3.,1.25000000000001,33.1));
#15482=CARTESIAN_POINT('',(10.,1.25000000000001,33.1));
#15483=CARTESIAN_POINT('Origin',(-3.,1.29111972369443E-14,33.1));
#15484=CARTESIAN_POINT('Origin',(10.,-7.778174593052,36.321825406948));
#15485=CARTESIAN_POINT('',(0.,-6.52817459305201,36.321825406948));
#15486=CARTESIAN_POINT('Origin',(0.,-7.77817459305201,36.321825406948));
#15487=CARTESIAN_POINT('',(-3.,-6.52817459305201,36.321825406948));
#15488=CARTESIAN_POINT('',(10.,-6.52817459305201,36.321825406948));
#15489=CARTESIAN_POINT('Origin',(-3.,-7.77817459305201,36.321825406948));
#15490=CARTESIAN_POINT('Origin',(10.,-11.,44.1));
#15491=CARTESIAN_POINT('',(0.,-9.74999999999998,44.1));
#15492=CARTESIAN_POINT('Origin',(0.,-11.,44.1));
#15493=CARTESIAN_POINT('',(-3.,-9.74999999999998,44.1));
#15494=CARTESIAN_POINT('',(10.,-9.74999999999998,44.1));
#15495=CARTESIAN_POINT('Origin',(-3.,-11.,44.1));
#15496=CARTESIAN_POINT('Origin',(10.,-7.778174593052,51.878174593052));
#15497=CARTESIAN_POINT('',(0.,-6.52817459305201,51.878174593052));
#15498=CARTESIAN_POINT('Origin',(0.,-7.77817459305201,51.878174593052));
#15499=CARTESIAN_POINT('',(-3.,-6.52817459305201,51.878174593052));
#15500=CARTESIAN_POINT('',(10.,-6.52817459305201,51.878174593052));
#15501=CARTESIAN_POINT('Origin',(-3.,-7.77817459305201,51.878174593052));
#15502=CARTESIAN_POINT('Origin',(10.,1.79671181153702E-14,55.1));
#15503=CARTESIAN_POINT('',(0.,1.25000000000001,55.1));
#15504=CARTESIAN_POINT('Origin',(0.,1.47451495458029E-14,55.1));
#15505=CARTESIAN_POINT('',(-3.,1.25000000000001,55.1));
#15506=CARTESIAN_POINT('',(10.,1.25000000000002,55.1));
#15507=CARTESIAN_POINT('Origin',(-3.,1.37785589749327E-14,55.1));
#15508=CARTESIAN_POINT('Origin',(10.,7.77817459305203,51.878174593052));
#15509=CARTESIAN_POINT('',(0.,9.02817459305204,51.878174593052));
#15510=CARTESIAN_POINT('Origin',(0.,7.77817459305203,51.878174593052));
#15511=CARTESIAN_POINT('',(-3.,9.02817459305203,51.878174593052));
#15512=CARTESIAN_POINT('',(10.,9.02817459305204,51.878174593052));
#15513=CARTESIAN_POINT('Origin',(-3.,7.77817459305203,51.878174593052));
#15514=CARTESIAN_POINT('Origin',(10.,11.,44.1));
#15515=CARTESIAN_POINT('',(0.,12.25,44.1));
#15516=CARTESIAN_POINT('Origin',(0.,11.,44.1));
#15517=CARTESIAN_POINT('',(-3.,12.25,44.1));
#15518=CARTESIAN_POINT('',(10.,12.25,44.1));
#15519=CARTESIAN_POINT('Origin',(-3.,11.,44.1));
#15520=CARTESIAN_POINT('Origin',(10.,4.95669204554415E-15,44.1));
#15521=CARTESIAN_POINT('',(0.,5.,44.1));
#15522=CARTESIAN_POINT('Origin',(0.,1.73472347597681E-15,44.1));
#15523=CARTESIAN_POINT('',(-3.,5.,44.1));
#15524=CARTESIAN_POINT('',(10.,5.,44.1));
#15525=CARTESIAN_POINT('Origin',(-3.,7.68132905106604E-16,44.1));
#15526=CARTESIAN_POINT('Origin',(0.,14.,88.2));
#15527=CARTESIAN_POINT('',(0.,14.,88.2));
#15528=CARTESIAN_POINT('',(-3.,14.,88.2));
#15529=CARTESIAN_POINT('',(0.,14.,88.2));
#15530=CARTESIAN_POINT('',(3.,17.,88.2));
#15531=CARTESIAN_POINT('Origin',(3.,14.,88.2));
#15532=CARTESIAN_POINT('',(3.,20.,88.2));
#15533=CARTESIAN_POINT('',(3.,20.,88.2));
#15534=CARTESIAN_POINT('Origin',(3.,14.,88.2));
#15535=CARTESIAN_POINT('Origin',(3.,20.,88.2));
#15536=CARTESIAN_POINT('',(4.51075599739428E-15,-14.,88.2));
#15537=CARTESIAN_POINT('',(0.,0.,88.2));
#15538=CARTESIAN_POINT('',(-3.,-14.,88.2));
#15539=CARTESIAN_POINT('',(-3.,0.,88.2));
#15540=CARTESIAN_POINT('',(-3.,-14.,88.2));
#15541=CARTESIAN_POINT('Origin',(3.,17.,0.));
#15542=CARTESIAN_POINT('',(3.,17.,0.));
#15543=CARTESIAN_POINT('',(3.,20.,0.));
#15544=CARTESIAN_POINT('',(3.,17.,0.));
#15545=CARTESIAN_POINT('',(0.,14.,0.));
#15546=CARTESIAN_POINT('Origin',(3.,14.,0.));
#15547=CARTESIAN_POINT('',(-3.,14.,0.));
#15548=CARTESIAN_POINT('',(-3.,14.,0.));
#15549=CARTESIAN_POINT('Origin',(3.,14.,0.));
#15550=CARTESIAN_POINT('Origin',(-3.,14.,0.));
#15551=CARTESIAN_POINT('',(3.96446609406726,20.,0.));
#15552=CARTESIAN_POINT('',(0.,20.,0.));
#15553=CARTESIAN_POINT('',(3.96446609406726,17.,0.));
#15554=CARTESIAN_POINT('',(3.96446609406726,14.,0.));
#15555=CARTESIAN_POINT('',(0.,17.,0.));
#15556=CARTESIAN_POINT('Origin',(3.,-17.,88.2));
#15557=CARTESIAN_POINT('',(3.,-17.,88.2));
#15558=CARTESIAN_POINT('',(3.,-20.,88.2));
#15559=CARTESIAN_POINT('',(3.,-17.,88.2));
#15560=CARTESIAN_POINT('Origin',(3.,-14.,88.2));
#15561=CARTESIAN_POINT('Origin',(3.,-14.,88.2));
#15562=CARTESIAN_POINT('Origin',(-3.,-14.,88.2));
#15563=CARTESIAN_POINT('',(3.96446609406726,-20.,88.2));
#15564=CARTESIAN_POINT('',(5.47734656826449E-15,-20.,88.2));
#15565=CARTESIAN_POINT('',(3.96446609406726,-17.,88.2));
#15566=CARTESIAN_POINT('',(3.96446609406726,-14.,88.2));
#15567=CARTESIAN_POINT('',(5.47734656826449E-15,-17.,88.2));
#15568=CARTESIAN_POINT('Origin',(4.51075599739428E-15,-14.,0.));
#15569=CARTESIAN_POINT('',(4.51075599739428E-15,-14.,0.));
#15570=CARTESIAN_POINT('',(-3.,-14.,0.));
#15571=CARTESIAN_POINT('',(4.51075599739428E-15,-14.,0.));
#15572=CARTESIAN_POINT('',(3.,-17.,0.));
#15573=CARTESIAN_POINT('Origin',(3.,-14.,0.));
#15574=CARTESIAN_POINT('',(3.,-20.,0.));
#15575=CARTESIAN_POINT('',(3.,-20.,0.));
#15576=CARTESIAN_POINT('Origin',(3.,-14.,0.));
#15577=CARTESIAN_POINT('Origin',(3.,-20.,0.));
#15578=CARTESIAN_POINT('',(0.,0.,0.));
#15579=CARTESIAN_POINT('',(-3.,-9.66590570870203E-16,0.));
#15580=CARTESIAN_POINT('Origin',(5.47734656826449E-15,-20.,88.2));
#15581=CARTESIAN_POINT('',(9.26776695296637,-20.,83.9322330470336));
#15582=CARTESIAN_POINT('',(5.73223304703362,-20.,87.4677669529664));
#15583=CARTESIAN_POINT('',(10.,-20.,83.2));
#15584=CARTESIAN_POINT('Origin',(3.96446609406726,-20.,85.7));
#15585=CARTESIAN_POINT('',(3.,-20.,88.2));
#15586=CARTESIAN_POINT('',(3.96446609406726,-20.,0.));
#15587=CARTESIAN_POINT('',(5.47734656826449E-15,-20.,0.));
#15588=CARTESIAN_POINT('',(5.73223304703363,-20.,0.732233047033637));
#15589=CARTESIAN_POINT('Origin',(3.96446609406726,-20.,2.5));
#15590=CARTESIAN_POINT('',(9.26776695296638,-20.,4.2677669529664));
#15591=CARTESIAN_POINT('',(5.,-20.,0.));
#15592=CARTESIAN_POINT('',(10.,-20.,6.03553390593277));
#15593=CARTESIAN_POINT('Origin',(7.5,-20.,6.03553390593277));
#15594=CARTESIAN_POINT('',(10.,-20.,82.1644660940673));
#15595=CARTESIAN_POINT('',(10.,-20.,88.2));
#15596=CARTESIAN_POINT('Origin',(7.5,-20.,82.1644660940673));
#15597=CARTESIAN_POINT('Origin',(10.,-17.,88.2));
#15598=CARTESIAN_POINT('',(10.,-17.,82.1644660940673));
#15599=CARTESIAN_POINT('',(10.,-17.,6.03553390593277));
#15600=CARTESIAN_POINT('',(10.,-17.,88.2));
#15601=CARTESIAN_POINT('',(10.,-17.,82.1644660940673));
#15602=CARTESIAN_POINT('',(10.,-17.,6.03553390593277));
#15603=CARTESIAN_POINT('Origin',(5.47734656826449E-15,-17.,88.2));
#15604=CARTESIAN_POINT('',(5.73223304703363,-17.,87.4677669529664));
#15605=CARTESIAN_POINT('Origin',(3.96446609406726,-17.,85.7));
#15606=CARTESIAN_POINT('',(9.26776695296638,-17.,83.9322330470336));
#15607=CARTESIAN_POINT('',(2.49999999999999,-17.,90.7));
#15608=CARTESIAN_POINT('Origin',(7.5,-17.,82.1644660940673));
#15609=CARTESIAN_POINT('',(9.26776695296638,-17.,4.2677669529664));
#15610=CARTESIAN_POINT('Origin',(7.5,-17.,6.03553390593277));
#15611=CARTESIAN_POINT('',(5.73223304703364,-17.,0.73223304703364));
#15612=CARTESIAN_POINT('',(46.6,-17.,41.6000000000003));
#15613=CARTESIAN_POINT('',(3.96446609406726,-17.,0.));
#15614=CARTESIAN_POINT('Origin',(3.96446609406726,-17.,2.5));
#15615=CARTESIAN_POINT('',(5.47734656826449E-15,-17.,0.));
#15616=CARTESIAN_POINT('',(3.,-17.,88.2));
#15617=CARTESIAN_POINT('Origin',(3.,-14.,88.2));
#15618=CARTESIAN_POINT('',(4.51075599739428E-15,-14.,88.2));
#15619=CARTESIAN_POINT('Origin',(0.,0.,88.2));
#15620=CARTESIAN_POINT('',(0.,14.,88.2));
#15621=CARTESIAN_POINT('Origin',(3.,14.,88.2));
#15622=CARTESIAN_POINT('',(3.,17.,88.2));
#15623=CARTESIAN_POINT('Origin',(0.,17.,88.2));
#15624=CARTESIAN_POINT('',(5.73223304703363,17.,0.732233047033647));
#15625=CARTESIAN_POINT('Origin',(3.96446609406726,17.,2.5));
#15626=CARTESIAN_POINT('',(9.26776695296638,17.,4.26776695296641));
#15627=CARTESIAN_POINT('',(46.6,17.,41.6000000000003));
#15628=CARTESIAN_POINT('',(10.,17.,6.03553390593277));
#15629=CARTESIAN_POINT('Origin',(7.5,17.,6.03553390593277));
#15630=CARTESIAN_POINT('',(10.,17.,82.1644660940673));
#15631=CARTESIAN_POINT('',(10.,17.,88.2));
#15632=CARTESIAN_POINT('',(9.26776695296637,17.,83.9322330470337));
#15633=CARTESIAN_POINT('Origin',(7.5,17.,82.1644660940673));
#15634=CARTESIAN_POINT('',(5.73223304703364,17.,87.4677669529664));
#15635=CARTESIAN_POINT('',(2.5,17.,90.7));
#15636=CARTESIAN_POINT('',(3.96446609406727,17.,88.2));
#15637=CARTESIAN_POINT('Origin',(3.96446609406727,17.,85.7));
#15638=CARTESIAN_POINT('',(0.,17.,88.2));
#15639=CARTESIAN_POINT('Origin',(10.,20.,88.2));
#15640=CARTESIAN_POINT('',(10.,20.,6.03553390593277));
#15641=CARTESIAN_POINT('',(10.,20.,6.03553390593277));
#15642=CARTESIAN_POINT('',(10.,20.,82.1644660940673));
#15643=CARTESIAN_POINT('',(10.,20.,88.2));
#15644=CARTESIAN_POINT('',(10.,20.,82.1644660940673));
#15645=CARTESIAN_POINT('Origin',(0.,20.,88.2));
#15646=CARTESIAN_POINT('',(9.26776695296638,20.,4.2677669529664));
#15647=CARTESIAN_POINT('',(5.73223304703363,20.,0.732233047033636));
#15648=CARTESIAN_POINT('',(5.,20.,0.));
#15649=CARTESIAN_POINT('Origin',(3.96446609406726,20.,2.5));
#15650=CARTESIAN_POINT('',(3.,20.,88.2));
#15651=CARTESIAN_POINT('',(3.96446609406727,20.,88.2));
#15652=CARTESIAN_POINT('',(0.,20.,88.2));
#15653=CARTESIAN_POINT('',(5.73223304703364,20.,87.4677669529664));
#15654=CARTESIAN_POINT('Origin',(3.96446609406727,20.,85.7));
#15655=CARTESIAN_POINT('',(9.26776695296637,20.,83.9322330470337));
#15656=CARTESIAN_POINT('',(10.,20.,83.2));
#15657=CARTESIAN_POINT('Origin',(7.5,20.,82.1644660940673));
#15658=CARTESIAN_POINT('Origin',(7.5,20.,6.03553390593277));
#15659=CARTESIAN_POINT('Origin',(3.,14.,88.2));
#15660=CARTESIAN_POINT('',(-3.,14.,88.2));
#15661=CARTESIAN_POINT('Origin',(-3.,-9.66590570870203E-16,88.2));
#15662=CARTESIAN_POINT('',(-3.,-14.,88.2));
#15663=CARTESIAN_POINT('Origin',(3.,-14.,88.2));
#15664=CARTESIAN_POINT('Origin',(3.,-14.,88.2));
#15665=CARTESIAN_POINT('',(3.96446609406727,20.,88.2));
#15666=CARTESIAN_POINT('Origin',(3.,-14.,0.));
#15667=CARTESIAN_POINT('',(3.96446609406726,-14.,0.));
#15668=CARTESIAN_POINT('Origin',(5.,-14.,0.));
#15669=CARTESIAN_POINT('',(9.26776695296638,-14.,4.2677669529664));
#15670=CARTESIAN_POINT('',(5.73223304703363,-14.,0.732233047033636));
#15671=CARTESIAN_POINT('Origin',(5.,14.,0.));
#15672=CARTESIAN_POINT('',(5.73223304703363,14.,0.732233047033636));
#15673=CARTESIAN_POINT('',(9.26776695296638,14.,4.2677669529664));
#15674=CARTESIAN_POINT('Origin',(10.,-17.,83.2));
#15675=CARTESIAN_POINT('',(5.73223304703363,-17.,87.4677669529664));
#15676=CARTESIAN_POINT('',(9.26776695296637,-17.,83.9322330470336));
#15677=CARTESIAN_POINT('Origin',(10.,20.,83.2));
#15678=CARTESIAN_POINT('',(5.73223304703364,17.,87.4677669529664));
#15679=CARTESIAN_POINT('',(9.26776695296637,20.,83.9322330470337));
#15680=CARTESIAN_POINT('Origin',(3.96446609406726,-14.,85.7));
#15681=CARTESIAN_POINT('Origin',(7.5,-17.,82.1644660940673));
#15682=CARTESIAN_POINT('Origin',(7.5,-17.,6.03553390593277));
#15683=CARTESIAN_POINT('Origin',(3.96446609406726,-14.,2.5));
#15684=CARTESIAN_POINT('Origin',(3.96446609406726,14.,2.5));
#15685=CARTESIAN_POINT('Origin',(7.5,20.,6.03553390593277));
#15686=CARTESIAN_POINT('Origin',(3.96446609406727,-14.,85.7));
#15687=CARTESIAN_POINT('Origin',(7.5,20.,82.1644660940673));
#20146=UNCERTAINTY_MEASURE_WITH_UNIT(LENGTH_MEASURE(0.01),#20177,
'DISTANCE_ACCURACY_VALUE',
'Maximum model space distance between geometric entities at asserted c
onnectivities');
#20160=UNCERTAINTY_MEASURE_WITH_UNIT(LENGTH_MEASURE(0.01),#20177,
'DISTANCE_ACCURACY_VALUE',
'Maximum model space distance between geometric entities at asserted c
onnectivities');
#20162=(
GEOMETRIC_REPRESENTATION_CONTEXT(3)
GLOBAL_UNCERTAINTY_ASSIGNED_CONTEXT((#20146))
GLOBAL_UNIT_ASSIGNED_CONTEXT((#20177,#20179,#20180))
REPRESENTATION_CONTEXT('','3D')
);
#20176=(
GEOMETRIC_REPRESENTATION_CONTEXT(3)
GLOBAL_UNCERTAINTY_ASSIGNED_CONTEXT((#20160))
GLOBAL_UNIT_ASSIGNED_CONTEXT((#20177,#20179,#20180))
REPRESENTATION_CONTEXT('','3D')
);
#20177=(
LENGTH_UNIT()
NAMED_UNIT(*)
SI_UNIT(.MILLI.,.METRE.)
);
#20179=(
NAMED_UNIT(*)
PLANE_ANGLE_UNIT()
SI_UNIT($,.RADIAN.)
);
#20180=(
NAMED_UNIT(*)
SI_UNIT($,.STERADIAN.)
SOLID_ANGLE_UNIT()
);
#20182=SHAPE_DEFINITION_REPRESENTATION(#20197,#20256);
#20197=PRODUCT_DEFINITION_SHAPE('',$,#20272);
#20256=SHAPE_REPRESENTATION('',(#11105),#20162);
#20270=PRODUCT_DEFINITION_CONTEXT('part definition',#20317,'design');
#20272=PRODUCT_DEFINITION('Double Bracket','Double Bracket',#20287,#20270);
#20287=PRODUCT_DEFINITION_FORMATION('',$,#20320);
#20317=APPLICATION_CONTEXT(
'Core Data for Automotive Mechanical Design Process');
#20318=PRODUCT_CONTEXT('part definition',#20317,'mechanical');
#20320=PRODUCT('Double Bracket','Double Bracket',$,(#20318));
#20335=PRESENTATION_STYLE_ASSIGNMENT((#20340));
#20340=SURFACE_STYLE_USAGE(.BOTH.,#20345);
#20345=SURFACE_SIDE_STYLE('',(#20350));
#20350=SURFACE_STYLE_FILL_AREA(#20355);
#20355=FILL_AREA_STYLE('Opaque(20,51,87)',(#20360));
#20360=FILL_AREA_STYLE_COLOUR('Opaque(20,51,87)',#20365);
#20365=COLOUR_RGB('Opaque(20,51,87)',0.0784313725490196,0.2,0.341176470588235);
ENDSEC;
END-ISO-10303-21;
